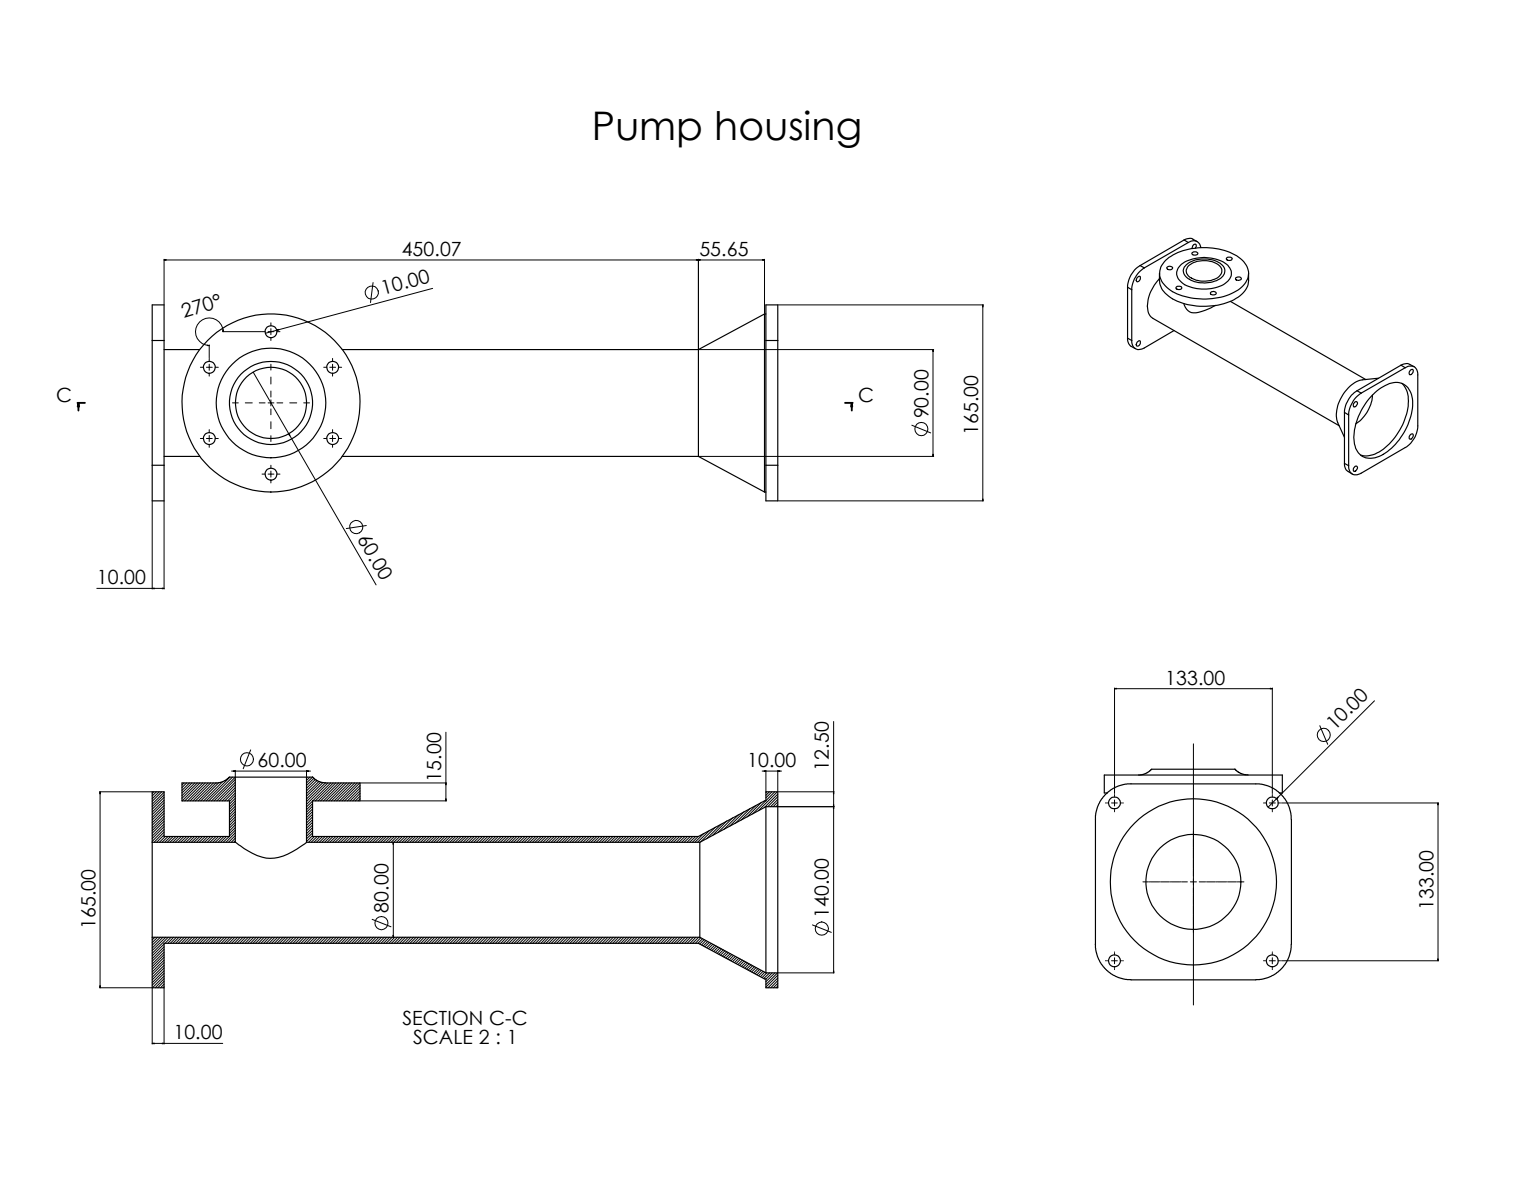
ISO-10303-21;
HEADER;
FILE_DESCRIPTION (('STEP AP214'),
    '1' );
FILE_NAME ('Pump housing.step',
    '2026-10-27T19:20:31',
    ( '' ),
    ( '' ),
    'SwSTEP 2.0',
    'SolidWorks 2025',
    '' );
FILE_SCHEMA (( 'AUTOMOTIVE_DESIGN' ));
ENDSEC;

DATA;
#8=( GEOMETRIC_REPRESENTATION_CONTEXT ( 3 ) GLOBAL_UNCERTAINTY_ASSIGNED_CONTEXT ( ( #20296 ) ) GLOBAL_UNIT_ASSIGNED_CONTEXT ( ( #22388, #16248, #14122 ) ) REPRESENTATION_CONTEXT ( 'NONE', 'WORKASPACE' ) );
#9=CARTESIAN_POINT ( 'NONE',  ( -200.0000000000000000, -52.49999999999992895, -52.49999999999999289 ) ) ;
#18=LINE ( 'NONE', #3258, #24208 ) ;
#20=CARTESIAN_POINT ( 'NONE',  ( -678.9461782662772293, 90.00000000000000000, 30.00000000000158096 ) ) ;
#22=DIRECTION ( 'NONE',  ( 0.000000000000000000, 0.000000000000000000, 1.000000000000000000 ) ) ;
#24=ORIENTED_EDGE ( 'NONE', *, *, #545, .T. ) ;
#40=DIRECTION ( 'NONE',  ( 0.000000000000000000, -0.000000000000000000, 1.000000000000000000 ) ) ;
#68=CARTESIAN_POINT ( 'NONE',  ( -210.0000000000000284, -52.49999999999991473, 82.49999999999998579 ) ) ;
#87=VERTEX_POINT ( 'NONE', #1727 ) ;
#102=DIRECTION ( 'NONE',  ( -1.000000000000000000, -1.836970198721030181E-16, 0.000000000000000000 ) ) ;
#143=DIRECTION ( 'NONE',  ( 0.000000000000000000, 1.000000000000000000, 0.000000000000000000 ) ) ;
#144=DIRECTION ( 'NONE',  ( 0.000000000000000000, 0.000000000000000000, 1.000000000000000000 ) ) ;
#153=DIRECTION ( 'NONE',  ( 1.000000000000000000, -0.000000000000000000, -0.000000000000000000 ) ) ;
#158=ORIENTED_EDGE ( 'NONE', *, *, #24110, .F. ) ;
#160=LINE ( 'NONE', #12392, #2622 ) ;
#170=CARTESIAN_POINT ( 'NONE',  ( -654.9559990268497813, 38.50095308322672594, 10.88967829900012418 ) ) ;
#178=CYLINDRICAL_SURFACE ( 'NONE', #9570, 69.99999999999998579 ) ;
#187=EDGE_LOOP ( 'NONE', ( #24603, #23674, #1863, #22741 ) ) ;
#188=ORIENTED_EDGE ( 'NONE', *, *, #14494, .T. ) ;
#231=AXIS2_PLACEMENT_3D ( 'NONE', #20688, #10567, #468 ) ;
#243=ORIENTED_EDGE ( 'NONE', *, *, #21209, .F. ) ;
#246=AXIS2_PLACEMENT_3D ( 'NONE', #22417, #6170, #12157 ) ;
#253=DIRECTION ( 'NONE',  ( 0.000000000000000000, 1.000000000000000000, 0.000000000000000000 ) ) ;
#254=DIRECTION ( 'NONE',  ( 0.000000000000000000, 0.000000000000000000, 1.000000000000000000 ) ) ;
#257=CIRCLE ( 'NONE', #21922, 30.00000000000000355 ) ;
#265=CIRCLE ( 'NONE', #15136, 44.99999999999997158 ) ;
#291=ADVANCED_FACE ( 'NONE', ( #12485 ), #392, .F. ) ;
#295=CIRCLE ( 'NONE', #24520, 34.99999999999999289 ) ;
#309=CARTESIAN_POINT ( 'NONE',  ( -655.7547062770219100, 39.08587256449166603, 8.516853268417087008 ) ) ;
#314=CIRCLE ( 'NONE', #24034, 5.000000000000011546 ) ;
#319=CARTESIAN_POINT ( 'NONE',  ( -661.6513161486427634, 44.74118846189777088, 4.856359999860261567 ) ) ;
#322=CIRCLE ( 'NONE', #24542, 5.000000000000004441 ) ;
#361=DIRECTION ( 'NONE',  ( 0.000000000000000000, 0.000000000000000000, 1.000000000000000000 ) ) ;
#383=ORIENTED_EDGE ( 'NONE', *, *, #7506, .F. ) ;
#392=CYLINDRICAL_SURFACE ( 'NONE', #8339, 5.000000000000007994 ) ;
#398=AXIS2_PLACEMENT_3D ( 'NONE', #8466, #22714, #5020 ) ;
#404=DIRECTION ( 'NONE',  ( 0.000000000000000000, 1.000000000000000000, 0.000000000000000000 ) ) ;
#408=LINE ( 'NONE', #4009, #2409 ) ;
#419=ORIENTED_EDGE ( 'NONE', *, *, #4206, .T. ) ;
#420=CARTESIAN_POINT ( 'NONE',  ( -726.9846540392142060, -66.50000000000001421, -66.50000000000005684 ) ) ;
#439=CIRCLE ( 'NONE', #14817, 44.99999999999997158 ) ;
#445=CARTESIAN_POINT ( 'NONE',  ( -650.6286843459992042, 35.47998694306583189, 18.48952057123083037 ) ) ;
#451=DIRECTION ( 'NONE',  ( 0.000000000000000000, 0.000000000000000000, -1.000000000000000000 ) ) ;
#455=CARTESIAN_POINT ( 'NONE',  ( -649.9764076924376468, 36.43131350046466821, 26.47907437413556053 ) ) ;
#462=DIRECTION ( 'NONE',  ( -1.000000000000000000, 0.000000000000000000, 0.000000000000000000 ) ) ;
#465=EDGE_CURVE ( 'NONE', #21399, #16736, #13986, .T. ) ;
#468=DIRECTION ( 'NONE',  ( 0.000000000000000000, 0.000000000000000000, 1.000000000000000000 ) ) ;
#472=DIRECTION ( 'NONE',  ( 0.000000000000000000, 0.000000000000000000, 1.000000000000000000 ) ) ;
#504=CARTESIAN_POINT ( 'NONE',  ( -726.9846540392142060, 52.49999999999986500, 82.49999999999998579 ) ) ;
#517=DIRECTION ( 'NONE',  ( 0.000000000000000000, 0.000000000000000000, 1.000000000000000000 ) ) ;
#526=DIRECTION ( 'NONE',  ( 0.000000000000000000, 0.000000000000000000, 1.000000000000000000 ) ) ;
#532=EDGE_CURVE ( 'NONE', #15801, #13855, #7476, .T. ) ;
#542=CARTESIAN_POINT ( 'NONE',  ( -597.4202930725263059, 39.67406997103029198, 5.193980993137010671 ) ) ;
#545=EDGE_CURVE ( 'NONE', #9566, #22711, #18550, .T. ) ;
#557=DIRECTION ( 'NONE',  ( 0.000000000000000000, 0.000000000000000000, 1.000000000000000000 ) ) ;
#567=VERTEX_POINT ( 'NONE', #26132 ) ;
#579=CARTESIAN_POINT ( 'NONE',  ( -656.5498746188114865, 39.67471111131991535, -5.189028119869940170 ) ) ;
#584=CARTESIAN_POINT ( 'NONE',  ( -265.6482238768269326, 0.000000000000000000, 0.000000000000000000 ) ) ;
#586=DIRECTION ( 'NONE',  ( 1.000000000000000000, 1.836970198721030427E-16, 0.000000000000000000 ) ) ;
#592=CARTESIAN_POINT ( 'NONE',  ( -611.2898122108906591, 32.33625437144371517, -31.30306668446011642 ) ) ;
#604=LINE ( 'NONE', #14430, #23210 ) ;
#609=DIRECTION ( 'NONE',  ( 0.000000000000000000, 0.000000000000000000, -1.000000000000000000 ) ) ;
#626=EDGE_CURVE ( 'NONE', #8935, #25083, #18123, .T. ) ;
#627=ORIENTED_EDGE ( 'NONE', *, *, #1350, .F. ) ;
#658=CARTESIAN_POINT ( 'NONE',  ( -678.9461782662772293, 75.00000000000000000, 35.00000000000159162 ) ) ;
#676=CARTESIAN_POINT ( 'NONE',  ( -716.9846540392142060, 66.50000000000009948, 61.50000000000005684 ) ) ;
#680=PLANE ( 'NONE',  #24960 ) ;
#685=FACE_OUTER_BOUND ( 'NONE', #11342, .T. ) ;
#687=EDGE_CURVE ( 'NONE', #14320, #23489, #997, .T. ) ;
#692=AXIS2_PLACEMENT_3D ( 'NONE', #22776, #2285, #14907 ) ;
#702=LINE ( 'NONE', #834, #8135 ) ;
#710=DIRECTION ( 'NONE',  ( 0.000000000000000000, 0.000000000000000000, -1.000000000000000000 ) ) ;
#713=DIRECTION ( 'NONE',  ( 0.000000000000000000, 0.000000000000000000, 1.000000000000000000 ) ) ;
#722=CARTESIAN_POINT ( 'NONE',  ( -661.7419054499291633, 44.81143869219462772, -4.158744080377950070 ) ) ;
#724=VECTOR ( 'NONE', #14723, 1000.000000000000000 ) ;
#728=CARTESIAN_POINT ( 'NONE',  ( -592.0657137250348114, 44.93697794005576185, -2.456499637838828853 ) ) ;
#740=CIRCLE ( 'NONE', #4985, 5.000000000000095035 ) ;
#749=DIRECTION ( 'NONE',  ( -1.000000000000000000, -1.836970198721030181E-16, 0.000000000000000000 ) ) ;
#758=ORIENTED_EDGE ( 'NONE', *, *, #3424, .F. ) ;
#770=DIRECTION ( 'NONE',  ( 0.000000000000000000, 1.000000000000000000, 0.000000000000000000 ) ) ;
#807=CARTESIAN_POINT ( 'NONE',  ( -617.0807177054949761, 28.23630110923742365, 28.33531756806318214 ) ) ;
#813=FACE_OUTER_BOUND ( 'NONE', #11620, .T. ) ;
#822=AXIS2_PLACEMENT_3D ( 'NONE', #9624, #3638, #5764 ) ;
#823=CARTESIAN_POINT ( 'NONE',  ( -678.9461782662789346, 90.00000000000000000, -24.99999999999826628 ) ) ;
#834=CARTESIAN_POINT ( 'NONE',  ( -678.9461782662772293, 75.00000000000000000, 25.00000000000157385 ) ) ;
#851=CARTESIAN_POINT ( 'NONE',  ( -642.7070543445415751, 32.34947999245193273, 31.28956669078001340 ) ) ;
#857=CARTESIAN_POINT ( 'NONE',  ( -592.4919920315402351, 44.60627086681392228, -6.055351194787411906 ) ) ;
#867=AXIS2_PLACEMENT_3D ( 'NONE', #5163, #9025, #21137 ) ;
#869=EDGE_CURVE ( 'NONE', #20514, #9693, #9078, .T. ) ;
#880=EDGE_CURVE ( 'NONE', #12353, #2322, #17250, .T. ) ;
#893=DIRECTION ( 'NONE',  ( -1.000000000000000000, -1.836970198721030181E-16, 0.000000000000000000 ) ) ;
#918=AXIS2_PLACEMENT_3D ( 'NONE', #25838, #19695, #3477 ) ;
#930=AXIS2_PLACEMENT_3D ( 'NONE', #26089, #1997, #5984 ) ;
#937=CARTESIAN_POINT ( 'NONE',  ( -605.2485198462496783, 34.24030537962636345, 20.68249523888561470 ) ) ;
#956=EDGE_LOOP ( 'NONE', ( #1715, #1989, #25855, #13026 ) ) ;
#958=CIRCLE ( 'NONE', #7716, 5.000000000000011546 ) ;
#978=LINE ( 'NONE', #16933, #23009 ) ;
#979=DIRECTION ( 'NONE',  ( 1.000000000000000000, -0.000000000000000000, -0.000000000000000000 ) ) ;
#987=CARTESIAN_POINT ( 'NONE',  ( -608.3670141342350917, 33.85940881687466231, 29.64264663930133992 ) ) ;
#997=B_SPLINE_CURVE_WITH_KNOTS ( 'NONE', 3,
 ( #7874, #1158, #13256, #1778, #9883, #26275, #12144, #15374, #24123, #5894, #14002, #10153, #20132, #21379, #25380, #22132, #21504, #3150, #7132, #15244, #23376, #12012, #5151, #11252, #19371, #3275, #9262, #17369, #25506, #7256, #23497, #579, #24530, #10410, #22405, #22927, #2713, #20665, #8149, #4438, #8686, #2301, #309, #6681, #170, #8411, #2177, #6159, #2573, #4708, #16264, #6418, #445, #4315, #24393, #16795, #12812, #18527, #12672, #18658, #4181, #16533, #18393, #8548, #14796, #10547, #6286, #12276, #20934, #24661, #14268, #18798, #14535, #22666 ),
 .UNSPECIFIED., .F., .F.,
 ( 4, 2, 2, 2, 2, 2, 2, 2, 2, 2, 2, 2, 2, 2, 2, 2, 2, 2, 2, 2, 2, 2, 2, 2, 2, 2, 2, 2, 2, 2, 2, 2, 2, 2, 2, 2, 4 ),
 ( 0.09798846907125773054, 0.09951654375267081354, 0.1010446184340838827, 0.1041007677969100348, 0.1071569171597361869, 0.1102130665225623529, 0.1132692158853885050, 0.1163253652482146572, 0.1224376639738672112, 0.1239657386552804053, 0.1254938133366935993, 0.1285499626995199873, 0.1346622614251727357, 0.1361903361065859297, 0.1377184107879991515, 0.1407745601508255950, 0.1438307095136520108, 0.1453587841950652049, 0.1468868588764783989, 0.1529991576021312305, 0.1545272322835444245, 0.1560553069649576186, 0.1591114563277840066, 0.1606395310091972561, 0.1621676056906105057, 0.1652237550534370325, 0.1682799044162635593, 0.1698079790976768089, 0.1713360537790900584, 0.1774483525047432786, 0.1805045018675699997, 0.1820325765489833603, 0.1835606512303967208, 0.1896729499560510512, 0.1927290993188783552, 0.1942571740002920211, 0.1957852486817056592 ),
 .UNSPECIFIED. ) ;
#1001=DIRECTION ( 'NONE',  ( -1.000000000000000000, 0.000000000000000000, 0.000000000000000000 ) ) ;
#1003=CARTESIAN_POINT ( 'NONE',  ( -626.9846540392142060, 90.00000000000000000, 0.000000000000000000 ) ) ;
#1004=LINE ( 'NONE', #19348, #9721 ) ;
#1045=ADVANCED_FACE ( 'NONE', ( #24084, #5858, #5998, #13964, #22099, #22760, #8115, #10649 ), #20625, .F. ) ;
#1079=ORIENTED_EDGE ( 'NONE', *, *, #14192, .F. ) ;
#1081=DIRECTION ( 'NONE',  ( -1.836970198721030427E-16, 1.000000000000000000, -1.321694076934715579E-16 ) ) ;
#1087=CARTESIAN_POINT ( 'NONE',  ( -716.9846540392142060, 66.50000000000009948, -61.50000000000004974 ) ) ;
#1089=CARTESIAN_POINT ( 'NONE',  ( -626.9846540392142060, 75.00000000000000000, -54.99999999999995026 ) ) ;
#1094=DIRECTION ( 'NONE',  ( 0.000000000000000000, 0.000000000000000000, 1.000000000000000000 ) ) ;
#1100=CARTESIAN_POINT ( 'NONE',  ( 0.000000000000000000, 0.000000000000000000, 0.000000000000000000 ) ) ;
#1103=AXIS2_PLACEMENT_3D ( 'NONE', #2737, #10842, #13228 ) ;
#1107=CARTESIAN_POINT ( 'NONE',  ( -626.9846540392142060, 75.00000000000000000, -65.00000000000004263 ) ) ;
#1116=CYLINDRICAL_SURFACE ( 'NONE', #8150, 44.99999999999997158 ) ;
#1118=EDGE_LOOP ( 'NONE', ( #10707, #11181, #17708, #25036 ) ) ;
#1123=CIRCLE ( 'NONE', #20660, 39.99999999999997158 ) ;
#1126=EDGE_CURVE ( 'NONE', #8002, #9153, #408, .T. ) ;
#1139=LINE ( 'NONE', #17860, #8300 ) ;
#1145=AXIS2_PLACEMENT_3D ( 'NONE', #16360, #16231, #22372 ) ;
#1152=CIRCLE ( 'NONE', #8804, 29.99999999999999289 ) ;
#1158=CARTESIAN_POINT ( 'NONE',  ( -627.5027443299393326, 26.45751311064577038, -30.00000000000005329 ) ) ;
#1177=LINE ( 'NONE', #21004, #23952 ) ;
#1180=VERTEX_POINT ( 'NONE', #10214 ) ;
#1184=CARTESIAN_POINT ( 'NONE',  ( 0.000000000000000000, 0.000000000000000000, 0.000000000000000000 ) ) ;
#1188=DIRECTION ( 'NONE',  ( 1.000000000000000000, -0.000000000000000000, -0.000000000000000000 ) ) ;
#1193=CARTESIAN_POINT ( 'NONE',  ( -598.6670741908344553, 38.75362502970266121, -9.956152867874221712 ) ) ;
#1200=EDGE_CURVE ( 'NONE', #17385, #7220, #19400, .T. ) ;
#1202=ORIENTED_EDGE ( 'NONE', *, *, #1431, .T. ) ;
#1213=ORIENTED_EDGE ( 'NONE', *, *, #19964, .F. ) ;
#1239=FACE_OUTER_BOUND ( 'NONE', #12293, .T. ) ;
#1240=CARTESIAN_POINT ( 'NONE',  ( -614.3062485512364219, 30.98201105461428995, 32.64211941558109942 ) ) ;
#1266=DIRECTION ( 'NONE',  ( -1.000000000000000000, 0.000000000000000000, 0.000000000000000000 ) ) ;
#1274=FACE_OUTER_BOUND ( 'NONE', #4173, .T. ) ;
#1282=AXIS2_PLACEMENT_3D ( 'NONE', #20, #15834, #6140 ) ;
#1310=CARTESIAN_POINT ( 'NONE',  ( -626.9846540392142060, 75.00000000000000000, 0.000000000000000000 ) ) ;
#1315=CARTESIAN_POINT ( 'NONE',  ( -611.8146452038604366, 30.48906968622233649, -25.89952525135564798 ) ) ;
#1336=VERTEX_POINT ( 'NONE', #11014 ) ;
#1337=EDGE_CURVE ( 'NONE', #2862, #11180, #19124, .T. ) ;
#1338=VERTEX_POINT ( 'NONE', #8746 ) ;
#1343=AXIS2_PLACEMENT_3D ( 'NONE', #16929, #25063, #6815 ) ;
#1350=EDGE_CURVE ( 'NONE', #16014, #12649, #10884, .T. ) ;
#1366=CARTESIAN_POINT ( 'NONE',  ( -639.6467708969067871, 30.97534985185962242, -32.64842303514383559 ) ) ;
#1375=FACE_OUTER_BOUND ( 'NONE', #4952, .T. ) ;
#1386=DIRECTION ( 'NONE',  ( 1.000000000000000000, -0.000000000000000000, -0.000000000000000000 ) ) ;
#1398=DIRECTION ( 'NONE',  ( 0.000000000000000000, -1.000000000000000000, 0.000000000000000000 ) ) ;
#1401=ORIENTED_EDGE ( 'NONE', *, *, #19720, .F. ) ;
#1431=EDGE_CURVE ( 'NONE', #11418, #14640, #18510, .T. ) ;
#1432=ORIENTED_EDGE ( 'NONE', *, *, #16631, .F. ) ;
#1461=ORIENTED_EDGE ( 'NONE', *, *, #4114, .T. ) ;
#1463=DIRECTION ( 'NONE',  ( 1.000000000000000000, 1.836970198721030427E-16, -0.000000000000000000 ) ) ;
#1470=LINE ( 'NONE', #1089, #20851 ) ;
#1473=DIRECTION ( 'NONE',  ( 1.000000000000000000, -0.000000000000000000, -0.000000000000000000 ) ) ;
#1490=ORIENTED_EDGE ( 'NONE', *, *, #16234, .F. ) ;
#1492=EDGE_CURVE ( 'NONE', #12353, #7498, #10988, .T. ) ;
#1493=DIRECTION ( 'NONE',  ( -1.000000000000000000, -1.836970198721030181E-16, 0.000000000000000000 ) ) ;
#1494=CARTESIAN_POINT ( 'NONE',  ( -615.3642883616319068, 30.56114224079260211, 33.03453977807346575 ) ) ;
#1496=CARTESIAN_POINT ( 'NONE',  ( -265.6482238768269326, 4.898587196589409870E-15, 39.99999999999997158 ) ) ;
#1503=ORIENTED_EDGE ( 'NONE', *, *, #5754, .F. ) ;
#1515=DIRECTION ( 'NONE',  ( 0.000000000000000000, 0.000000000000000000, -1.000000000000000000 ) ) ;
#1529=ADVANCED_FACE ( 'NONE', ( #17473 ), #21477, .F. ) ;
#1531=EDGE_LOOP ( 'NONE', ( #6366, #4909, #3109, #25138 ) ) ;
#1533=VECTOR ( 'NONE', #12308, 1000.000000000000000 ) ;
#1548=AXIS2_PLACEMENT_3D ( 'NONE', #18108, #1759, #22118 ) ;
#1559=ORIENTED_EDGE ( 'NONE', *, *, #25834, .T. ) ;
#1564=VERTEX_POINT ( 'NONE', #25870 ) ;
#1586=CARTESIAN_POINT ( 'NONE',  ( -210.0000000000000284, 66.50000000000009948, 66.50000000000005684 ) ) ;
#1593=VERTEX_POINT ( 'NONE', #3641 ) ;
#1596=VERTEX_POINT ( 'NONE', #23600 ) ;
#1599=ORIENTED_EDGE ( 'NONE', *, *, #18731, .T. ) ;
#1601=DIRECTION ( 'NONE',  ( -1.000000000000000000, 0.000000000000000000, 0.000000000000000000 ) ) ;
#1630=ORIENTED_EDGE ( 'NONE', *, *, #20692, .F. ) ;
#1639=CARTESIAN_POINT ( 'NONE',  ( -210.0000000000000284, -61.50000000000002132, -66.50000000000005684 ) ) ;
#1651=CARTESIAN_POINT ( 'NONE',  ( -626.9846540392142060, 95.00000000000000000, 30.00000000000005329 ) ) ;
#1652=DIRECTION ( 'NONE',  ( -1.000000000000000000, -1.836970198721030181E-16, 0.000000000000000000 ) ) ;
#1668=EDGE_CURVE ( 'NONE', #12661, #21773, #1139, .T. ) ;
#1678=DIRECTION ( 'NONE',  ( 1.000000000000000000, -0.000000000000000000, -0.000000000000000000 ) ) ;
#1684=CARTESIAN_POINT ( 'NONE',  ( -210.0000000000000284, 66.50000000000009948, 66.50000000000005684 ) ) ;
#1692=ORIENTED_EDGE ( 'NONE', *, *, #20350, .T. ) ;
#1708=CARTESIAN_POINT ( 'NONE',  ( -604.5625608938773894, 34.67764305556000437, -19.95380784793596973 ) ) ;
#1715=ORIENTED_EDGE ( 'NONE', *, *, #626, .F. ) ;
#1721=VERTEX_POINT ( 'NONE', #26011 ) ;
#1727=CARTESIAN_POINT ( 'NONE',  ( -265.6482238768269326, 0.000000000000000000, -39.99999999999997158 ) ) ;
#1746=CARTESIAN_POINT ( 'NONE',  ( -716.9846540392142060, 52.49999999999991473, -82.49999999999998579 ) ) ;
#1753=EDGE_LOOP ( 'NONE', ( #10197, #3904, #12389, #11955 ) ) ;
#1757=CARTESIAN_POINT ( 'NONE',  ( -716.9846540392142060, 52.50000000000007816, -52.49999999999999289 ) ) ;
#1759=DIRECTION ( 'NONE',  ( 0.000000000000000000, 1.000000000000000000, 0.000000000000000000 ) ) ;
#1760=VERTEX_POINT ( 'NONE', #1651 ) ;
#1761=CIRCLE ( 'NONE', #7270, 30.00000000000000355 ) ;
#1767=ORIENTED_EDGE ( 'NONE', *, *, #12722, .F. ) ;
#1777=CYLINDRICAL_SURFACE ( 'NONE', #3646, 5.000000000000011546 ) ;
#1778=CARTESIAN_POINT ( 'NONE',  ( -629.0557304578984485, 26.53345902544097967, -29.93287798360601570 ) ) ;
#1797=ORIENTED_EDGE ( 'NONE', *, *, #5393, .F. ) ;
#1825=EDGE_LOOP ( 'NONE', ( #17662, #23179 ) ) ;
#1850=DIRECTION ( 'NONE',  ( 0.000000000000000000, -1.000000000000000000, 0.000000000000000000 ) ) ;
#1852=ORIENTED_EDGE ( 'NONE', *, *, #12545, .T. ) ;
#1863=ORIENTED_EDGE ( 'NONE', *, *, #1350, .T. ) ;
#1868=CARTESIAN_POINT ( 'NONE',  ( -726.9846540392142060, 66.50000000000009948, 61.50000000000005684 ) ) ;
#1880=DIRECTION ( 'NONE',  ( 0.000000000000000000, 1.000000000000000000, 0.000000000000000000 ) ) ;
#1890=DIRECTION ( 'NONE',  ( 0.000000000000000000, 0.000000000000000000, -1.000000000000000000 ) ) ;
#1895=( NAMED_UNIT ( * ) SI_UNIT ( $, .STERADIAN. ) SOLID_ANGLE_UNIT ( ) );
#1897=ORIENTED_EDGE ( 'NONE', *, *, #626, .T. ) ;
#1910=CARTESIAN_POINT ( 'NONE',  ( -626.9846540392142060, 75.00000000000000000, -74.99999999999991473 ) ) ;
#1916=DIRECTION ( 'NONE',  ( 0.000000000000000000, 0.000000000000000000, 1.000000000000000000 ) ) ;
#1921=CARTESIAN_POINT ( 'NONE',  ( -678.9461782662789346, 75.00000000000000000, -24.99999999999826628 ) ) ;
#1928=ORIENTED_EDGE ( 'NONE', *, *, #25834, .F. ) ;
#1955=AXIS2_PLACEMENT_3D ( 'NONE', #23408, #21788, #23653 ) ;
#1962=VECTOR ( 'NONE', #14925, 1000.000000000000000 ) ;
#1988=EDGE_LOOP ( 'NONE', ( #758, #21990, #4423, #14129 ) ) ;
#1989=ORIENTED_EDGE ( 'NONE', *, *, #16482, .T. ) ;
#1997=DIRECTION ( 'NONE',  ( -1.000000000000000000, 0.000000000000000000, 0.000000000000000000 ) ) ;
#2000=AXIS2_PLACEMENT_3D ( 'NONE', #23417, #23537, #25292 ) ;
#2019=LINE ( 'NONE', #4153, #21289 ) ;
#2030=DIRECTION ( 'NONE',  ( -1.000000000000000000, 0.000000000000000000, 0.000000000000000000 ) ) ;
#2041=CARTESIAN_POINT ( 'NONE',  ( -199.9999999999999716, -82.49999999999991473, -52.49999999999977973 ) ) ;
#2049=CARTESIAN_POINT ( 'NONE',  ( -716.9846540392142060, 82.50000000000008527, 52.49999999999980105 ) ) ;
#2054=LINE ( 'NONE', #16410, #18940 ) ;
#2064=ORIENTED_EDGE ( 'NONE', *, *, #22985, .T. ) ;
#2065=ORIENTED_EDGE ( 'NONE', *, *, #22233, .F. ) ;
#2077=LINE ( 'NONE', #4214, #17372 ) ;
#2081=LINE ( 'NONE', #16303, #1533 ) ;
#2094=ORIENTED_EDGE ( 'NONE', *, *, #16482, .F. ) ;
#2102=CARTESIAN_POINT ( 'NONE',  ( -575.0231298121445889, 75.00000000000000000, 29.99999999999825206 ) ) ;
#2118=PRODUCT_CONTEXT ( 'NONE', #10201, 'mechanical' ) ;
#2123=ORIENTED_EDGE ( 'NONE', *, *, #23092, .F. ) ;
#2139=DIRECTION ( 'NONE',  ( 1.000000000000000000, 1.836970198721030427E-16, -0.000000000000000000 ) ) ;
#2143=FACE_BOUND ( 'NONE', #4565, .T. ) ;
#2144=AXIS2_PLACEMENT_3D ( 'NONE', #13336, #11585, #19580 ) ;
#2152=VERTEX_POINT ( 'NONE', #16029 ) ;
#2154=FACE_OUTER_BOUND ( 'NONE', #25295, .T. ) ;
#2163=DIRECTION ( 'NONE',  ( 0.8802361161597900274, 0.000000000000000000, -0.4745359626076074422 ) ) ;
#2165=ADVANCED_FACE ( 'NONE', ( #7613 ), #14146, .F. ) ;
#2171=EDGE_CURVE ( 'NONE', #24112, #7498, #20193, .T. ) ;
#2172=ADVANCED_FACE ( 'NONE', ( #22935 ), #6425, .F. ) ;
#2177=CARTESIAN_POINT ( 'NONE',  ( -654.1659037529333318, 37.93148257888354635, 12.70525021040782754 ) ) ;
#2180=DIRECTION ( 'NONE',  ( -1.000000000000000000, 0.000000000000000000, 0.000000000000000000 ) ) ;
#2187=FACE_BOUND ( 'NONE', #25625, .T. ) ;
#2198=ORIENTED_EDGE ( 'NONE', *, *, #19384, .F. ) ;
#2204=FACE_OUTER_BOUND ( 'NONE', #13398, .T. ) ;
#2205=CARTESIAN_POINT ( 'NONE',  ( -726.9846540392142060, -52.49999999999991473, 82.49999999999998579 ) ) ;
#2227=DIRECTION ( 'NONE',  ( -1.000000000000000000, -1.836970198721030181E-16, 0.000000000000000000 ) ) ;
#2247=ORIENTED_EDGE ( 'NONE', *, *, #16442, .F. ) ;
#2252=EDGE_CURVE ( 'NONE', #6112, #5576, #6594, .T. ) ;
#2257=EDGE_LOOP ( 'NONE', ( #16312, #18069, #19048, #6656 ) ) ;
#2285=DIRECTION ( 'NONE',  ( -1.000000000000000000, 0.000000000000000000, 0.000000000000000000 ) ) ;
#2301=CARTESIAN_POINT ( 'NONE',  ( -655.8941833601360258, 39.18869065112085082, 8.031053782042897993 ) ) ;
#2311=CARTESIAN_POINT ( 'NONE',  ( -660.6855337863669320, 43.99654503343406020, 9.519970529664389502 ) ) ;
#2322=VERTEX_POINT ( 'NONE', #4715 ) ;
#2340=ADVANCED_FACE ( 'NONE', ( #12819 ), #178, .F. ) ;
#2387=VERTEX_POINT ( 'NONE', #24941 ) ;
#2404=EDGE_CURVE ( 'NONE', #1338, #2553, #2054, .T. ) ;
#2405=CARTESIAN_POINT ( 'NONE',  ( -716.9846540392142060, -52.49999999999992895, -52.49999999999999289 ) ) ;
#2409=VECTOR ( 'NONE', #2139, 1000.000000000000000 ) ;
#2410=FACE_OUTER_BOUND ( 'NONE', #20252, .T. ) ;
#2432=DIRECTION ( 'NONE',  ( 0.000000000000000000, 1.000000000000000000, 0.000000000000000000 ) ) ;
#2449=CARTESIAN_POINT ( 'NONE',  ( -592.4863246237233625, 44.61088836317698281, 5.935200987246425974 ) ) ;
#2453=DIRECTION ( 'NONE',  ( 0.000000000000000000, -1.000000000000000000, 0.000000000000000000 ) ) ;
#2482=ADVANCED_FACE ( 'NONE', ( #24803 ), #2580, .F. ) ;
#2499=DIRECTION ( 'NONE',  ( 0.000000000000000000, 1.000000000000000000, 0.000000000000000000 ) ) ;
#2518=ORIENTED_EDGE ( 'NONE', *, *, #3123, .F. ) ;
#2520=DIRECTION ( 'NONE',  ( 0.000000000000000000, 1.000000000000000000, 0.000000000000000000 ) ) ;
#2533=CARTESIAN_POINT ( 'NONE',  ( -598.0968614159205572, 39.17219949141968272, 8.155532079469960394 ) ) ;
#2546=DIRECTION ( 'NONE',  ( 0.000000000000000000, 0.000000000000000000, 1.000000000000000000 ) ) ;
#2548=AXIS2_PLACEMENT_3D ( 'NONE', #23606, #16375, #12123 ) ;
#2553=VERTEX_POINT ( 'NONE', #8910 ) ;
#2558=ORIENTED_EDGE ( 'NONE', *, *, #9614, .T. ) ;
#2568=DIRECTION ( 'NONE',  ( 0.000000000000000000, 1.000000000000000000, 0.000000000000000000 ) ) ;
#2573=CARTESIAN_POINT ( 'NONE',  ( -653.5054087259286462, 37.46094337825315534, 14.03175942970671386 ) ) ;
#2580=CYLINDRICAL_SURFACE ( 'NONE', #25729, 4.999999999999962697 ) ;
#2582=CARTESIAN_POINT ( 'NONE',  ( -653.4170159849278434, 38.71178713871361765, 22.94860588273028768 ) ) ;
#2587=CARTESIAN_POINT ( 'NONE',  ( -595.8093182457012063, 42.09229316366772622, 15.94989993472014511 ) ) ;
#2588=ORIENTED_EDGE ( 'NONE', *, *, #25417, .F. ) ;
#2592=DIRECTION ( 'NONE',  ( 1.000000000000000000, 1.836970198721030427E-16, -0.000000000000000000 ) ) ;
#2594=AXIS2_PLACEMENT_3D ( 'NONE', #23312, #23060, #22792 ) ;
#2597=DIRECTION ( 'NONE',  ( 0.000000000000000000, 0.000000000000000000, 1.000000000000000000 ) ) ;
#2609=CARTESIAN_POINT ( 'NONE',  ( -575.0231298121445889, 75.00000000000000000, 24.99999999999828759 ) ) ;
#2622=VECTOR ( 'NONE', #11998, 1000.000000000000000 ) ;
#2625=ORIENTED_EDGE ( 'NONE', *, *, #7357, .F. ) ;
#2664=AXIS2_PLACEMENT_3D ( 'NONE', #2981, #19204, #3354 ) ;
#2676=CARTESIAN_POINT ( 'NONE',  ( -619.9449226945228020, 27.37410191665372494, 29.16662018060867112 ) ) ;
#2694=FACE_BOUND ( 'NONE', #25987, .T. ) ;
#2696=ORIENTED_EDGE ( 'NONE', *, *, #3076, .F. ) ;
#2699=DIRECTION ( 'NONE',  ( 0.000000000000000000, 1.000000000000000000, 0.000000000000000000 ) ) ;
#2702=ORIENTED_EDGE ( 'NONE', *, *, #4106, .F. ) ;
#2713=CARTESIAN_POINT ( 'NONE',  ( -656.9835591184084933, 39.99917881009967147, -0.5754573772625048989 ) ) ;
#2722=CARTESIAN_POINT ( 'NONE',  ( -661.9203515605751136, 44.94993422606702893, 2.443437321343243429 ) ) ;
#2726=CARTESIAN_POINT ( 'NONE',  ( -595.8013259146971450, 42.09546181640034490, -16.06146874878389141 ) ) ;
#2733=ORIENTED_EDGE ( 'NONE', *, *, #6809, .T. ) ;
#2737=CARTESIAN_POINT ( 'NONE',  ( -210.0000000000000284, -52.49999999999991473, 52.49999999999999289 ) ) ;
#2751=ADVANCED_FACE ( 'NONE', ( #22759 ), #8510, .F. ) ;
#2754=DIRECTION ( 'NONE',  ( 0.000000000000000000, 0.000000000000000000, 1.000000000000000000 ) ) ;
#2765=CARTESIAN_POINT ( 'NONE',  ( 0.000000000000000000, 0.000000000000000000, -75.00000000000000000 ) ) ;
#2781=CYLINDRICAL_SURFACE ( 'NONE', #11057, 4.999999999999997335 ) ;
#2806=CARTESIAN_POINT ( 'NONE',  ( -622.8837209345899737, 26.70509413432482049, 29.78579685810782252 ) ) ;
#2809=AXIS2_PLACEMENT_3D ( 'NONE', #1003, #18966, #22694 ) ;
#2825=ORIENTED_EDGE ( 'NONE', *, *, #22824, .F. ) ;
#2842=EDGE_CURVE ( 'NONE', #5576, #15935, #17400, .T. ) ;
#2857=CIRCLE ( 'NONE', #22396, 15.00000000000000000 ) ;
#2858=ORIENTED_EDGE ( 'NONE', *, *, #9722, .F. ) ;
#2861=CARTESIAN_POINT ( 'NONE',  ( -603.9616649909638681, 36.45097493161564728, 26.45255915120217693 ) ) ;
#2862=VERTEX_POINT ( 'NONE', #15654 ) ;
#2864=DIRECTION ( 'NONE',  ( 0.000000000000000000, 1.000000000000000000, 0.000000000000000000 ) ) ;
#2867=ORIENTED_EDGE ( 'NONE', *, *, #19308, .F. ) ;
#2873=DIRECTION ( 'NONE',  ( -0.000000000000000000, 1.000000000000000000, -0.000000000000000000 ) ) ;
#2880=CARTESIAN_POINT ( 'NONE',  ( -200.0000000000000000, -66.50000000000001421, -66.50000000000005684 ) ) ;
#2899=EDGE_CURVE ( 'NONE', #2983, #16736, #10016, .T. ) ;
#2912=FACE_OUTER_BOUND ( 'NONE', #21555, .T. ) ;
#2915=VERTEX_POINT ( 'NONE', #23778 ) ;
#2942=ORIENTED_EDGE ( 'NONE', *, *, #9722, .T. ) ;
#2947=AXIS2_PLACEMENT_3D ( 'NONE', #6165, #26280, #1916 ) ;
#2950=EDGE_LOOP ( 'NONE', ( #17042, #10599, #1432, #9437 ) ) ;
#2951=EDGE_LOOP ( 'NONE', ( #2702, #19675, #20637, #14350 ) ) ;
#2962=LINE ( 'NONE', #21056, #3828 ) ;
#2970=ADVANCED_FACE ( 'NONE', ( #25664 ), #17526, .T. ) ;
#2971=VECTOR ( 'NONE', #12257, 1000.000000000000000 ) ;
#2976=CARTESIAN_POINT ( 'NONE',  ( -645.5897708877611194, 33.84656210914351959, -29.66564330929828230 ) ) ;
#2981=CARTESIAN_POINT ( 'NONE',  ( -716.9846540392142060, -66.50000000000001421, 66.50000000000005684 ) ) ;
#2982=CARTESIAN_POINT ( 'NONE',  ( -596.9048215538962268, 41.27960141593418797, -18.03334258849684701 ) ) ;
#2983=VERTEX_POINT ( 'NONE', #7410 ) ;
#2987=ADVANCED_FACE ( 'NONE', ( #7162 ), #15524, .T. ) ;
#2988=CARTESIAN_POINT ( 'NONE',  ( 0.000000000000000000, 0.000000000000000000, 0.000000000000000000 ) ) ;
#2996=LINE ( 'NONE', #20826, #10015 ) ;
#3008=AXIS2_PLACEMENT_3D ( 'NONE', #5611, #15208, #23458 ) ;
#3020=DIRECTION ( 'NONE',  ( 0.000000000000000000, 0.000000000000000000, 1.000000000000000000 ) ) ;
#3030=CARTESIAN_POINT ( 'NONE',  ( 0.000000000000000000, 9.184850993605148733E-15, 75.00000000000000000 ) ) ;
#3038=VECTOR ( 'NONE', #12658, 1000.000000000000000 ) ;
#3045=EDGE_LOOP ( 'NONE', ( #5456, #12790, #12055, #22189 ) ) ;
#3057=CARTESIAN_POINT ( 'NONE',  ( -210.0000000000000284, 0.000000000000000000, 0.000000000000000000 ) ) ;
#3060=CARTESIAN_POINT ( 'NONE',  ( -599.0758207628625769, 38.45631679711321738, 11.01587919049791076 ) ) ;
#3068=CARTESIAN_POINT ( 'NONE',  ( -716.9846540392142060, 66.50000000000009948, -66.50000000000005684 ) ) ;
#3073=CYLINDRICAL_SURFACE ( 'NONE', #6053, 5.000000000000004441 ) ;
#3076=EDGE_CURVE ( 'NONE', #23087, #10307, #2081, .T. ) ;
#3080=EDGE_LOOP ( 'NONE', ( #9441, #19397, #23709, #22220 ) ) ;
#3092=CARTESIAN_POINT ( 'NONE',  ( -716.9846540392142060, -82.49999999999991473, -52.49999999999977973 ) ) ;
#3103=CARTESIAN_POINT ( 'NONE',  ( -638.5875168204022430, 30.55437902294503161, -33.04080401100450359 ) ) ;
#3108=CARTESIAN_POINT ( 'NONE',  ( -617.0039382655427289, 29.98920333220143419, 33.55165781079447385 ) ) ;
#3109=ORIENTED_EDGE ( 'NONE', *, *, #9480, .F. ) ;
#3113=VERTEX_POINT ( 'NONE', #16438 ) ;
#3117=CARTESIAN_POINT ( 'NONE',  ( 0.000000000000000000, 0.000000000000000000, -44.99999999999997158 ) ) ;
#3120=DIRECTION ( 'NONE',  ( 0.000000000000000000, 0.000000000000000000, 1.000000000000000000 ) ) ;
#3123=EDGE_CURVE ( 'NONE', #21007, #20921, #20037, .T. ) ;
#3150=CARTESIAN_POINT ( 'NONE',  ( -648.4009115869816924, 34.03803227582063329, -21.01344779086421255 ) ) ;
#3151=EDGE_CURVE ( 'NONE', #1593, #6964, #20646, .T. ) ;
#3157=DIRECTION ( 'NONE',  ( 1.000000000000000000, -0.000000000000000000, -0.000000000000000000 ) ) ;
#3167=VERTEX_POINT ( 'NONE', #14039 ) ;
#3172=EDGE_LOOP ( 'NONE', ( #6273, #9609 ) ) ;
#3184=CARTESIAN_POINT ( 'NONE',  ( -598.2148974052754511, 39.08565501426862454, -8.517844816818030296 ) ) ;
#3203=CIRCLE ( 'NONE', #231, 5.000000000000039080 ) ;
#3224=AXIS2_PLACEMENT_3D ( 'NONE', #4997, #18960, #3120 ) ;
#3228=DIRECTION ( 'NONE',  ( -1.000000000000000000, 0.000000000000000000, 0.000000000000000000 ) ) ;
#3233=EDGE_LOOP ( 'NONE', ( #18372, #13913, #1559, #22423 ) ) ;
#3236=DIRECTION ( 'NONE',  ( -1.000000000000000000, -1.836970198721030181E-16, 0.000000000000000000 ) ) ;
#3238=ORIENTED_EDGE ( 'NONE', *, *, #25270, .F. ) ;
#3242=DIRECTION ( 'NONE',  ( 1.000000000000000000, 1.836970198721030427E-16, -0.000000000000000000 ) ) ;
#3243=CLOSED_SHELL ( 'NONE', ( #11757, #22727, #20867, #12476, #10434, #24263, #18492, #1529, #17565, #25370, #17208, #15951, #19396, #10881, #11280, #23525, #18081, #23913, #20057, #3963, #2165, #20870, #12486, #18771, #24445, #5556, #12232, #14264, #14679, #12482, #25042, #20355, #2970, #9287, #20548, #2172, #2987, #2751, #2340, #16882, #17246, #24951, #21636, #15474, #13245, #14824, #11974, #22263, #19247, #1045, #5863, #291, #2482, #7282, #5025, #6375, #9946, #4875, #5328, #14432, #8067, #4219, #9376, #10598, #17893, #12575, #9237, #14345, #24209, #24635, #22975 ) ) ;
#3244=DIRECTION ( 'NONE',  ( 0.000000000000000000, 0.000000000000000000, -1.000000000000000000 ) ) ;
#3258=CARTESIAN_POINT ( 'NONE',  ( -716.9846540392142060, -82.49999999999991473, 52.49999999999977263 ) ) ;
#3275=CARTESIAN_POINT ( 'NONE',  ( -654.7090520960496178, 38.32262798275520055, -11.47173633207906107 ) ) ;
#3312=CARTESIAN_POINT ( 'NONE',  ( -614.8060072283433328, 29.12309729869464192, -27.42103544326355546 ) ) ;
#3328=CARTESIAN_POINT ( 'NONE',  ( -678.9461782662772293, 75.00000000000000000, 30.00000000000158096 ) ) ;
#3330=ORIENTED_EDGE ( 'NONE', *, *, #18880, .T. ) ;
#3337=CARTESIAN_POINT ( 'NONE',  ( -210.0000000000000284, 0.000000000000000000, -75.00000000000000000 ) ) ;
#3345=AXIS2_PLACEMENT_3D ( 'NONE', #7445, #17435, #11438 ) ;
#3354=DIRECTION ( 'NONE',  ( 0.000000000000000000, 0.000000000000000000, 1.000000000000000000 ) ) ;
#3356=EDGE_LOOP ( 'NONE', ( #20075, #16422, #24649, #24167 ) ) ;
#3363=EDGE_CURVE ( 'NONE', #5576, #6112, #18528, .T. ) ;
#3378=DIRECTION ( 'NONE',  ( -1.000000000000000000, 0.000000000000000000, 0.000000000000000000 ) ) ;
#3390=AXIS2_PLACEMENT_3D ( 'NONE', #10930, #24638, #6792 ) ;
#3398=CYLINDRICAL_SURFACE ( 'NONE', #20716, 74.99999999999991473 ) ;
#3410=FACE_OUTER_BOUND ( 'NONE', #2257, .T. ) ;
#3415=ORIENTED_EDGE ( 'NONE', *, *, #11169, .T. ) ;
#3424=EDGE_CURVE ( 'NONE', #13855, #17045, #25460, .T. ) ;
#3425=CARTESIAN_POINT ( 'NONE',  ( -626.9846540392142060, 75.00000000000000000, 34.99999999999999289 ) ) ;
#3427=EDGE_CURVE ( 'NONE', #24064, #13093, #257, .T. ) ;
#3428=FACE_OUTER_BOUND ( 'NONE', #4333, .T. ) ;
#3434=CYLINDRICAL_SURFACE ( 'NONE', #13021, 29.99999999999999645 ) ;
#3435=CARTESIAN_POINT ( 'NONE',  ( -622.8776819133570370, 26.70401283558588901, -29.78701626806179092 ) ) ;
#3439=AXIS2_PLACEMENT_3D ( 'NONE', #18849, #2227, #25239 ) ;
#3442=AXIS2_PLACEMENT_3D ( 'NONE', #9692, #3450, #25808 ) ;
#3444=AXIS2_PLACEMENT_3D ( 'NONE', #3731, #1473, #7571 ) ;
#3450=DIRECTION ( 'NONE',  ( -1.000000000000000000, -1.836970198721030181E-16, 0.000000000000000000 ) ) ;
#3455=DIRECTION ( 'NONE',  ( 1.000000000000000000, 1.836970198721030427E-16, -0.000000000000000000 ) ) ;
#3463=CARTESIAN_POINT ( 'NONE',  ( -210.0000000000000284, 82.50000000000008527, -52.49999999999978684 ) ) ;
#3477=DIRECTION ( 'NONE',  ( 0.000000000000000000, 0.000000000000000000, -1.000000000000000000 ) ) ;
#3500=AXIS2_PLACEMENT_3D ( 'NONE', #9344, #7214, #17198 ) ;
#3520=ORIENTED_EDGE ( 'NONE', *, *, #10207, .F. ) ;
#3527=CARTESIAN_POINT ( 'NONE',  ( -716.9846540392142060, 52.49999999999986500, 82.49999999999998579 ) ) ;
#3557=CARTESIAN_POINT ( 'NONE',  ( -626.9846540392142060, 75.00000000000000000, -60.00000000000000000 ) ) ;
#3571=VERTEX_POINT ( 'NONE', #11332 ) ;
#3578=VERTEX_POINT ( 'NONE', #23331 ) ;
#3579=FACE_OUTER_BOUND ( 'NONE', #18647, .T. ) ;
#3581=ORIENTED_EDGE ( 'NONE', *, *, #17434, .T. ) ;
#3626=EDGE_CURVE ( 'NONE', #17304, #7651, #19784, .T. ) ;
#3635=DIRECTION ( 'NONE',  ( 0.000000000000000000, 0.000000000000000000, 1.000000000000000000 ) ) ;
#3638=DIRECTION ( 'NONE',  ( -1.000000000000000000, -1.836970198721030181E-16, 0.000000000000000000 ) ) ;
#3641=CARTESIAN_POINT ( 'NONE',  ( -716.9846540392142060, -66.50000000000001421, -71.50000000000005684 ) ) ;
#3646=AXIS2_PLACEMENT_3D ( 'NONE', #3911, #15850, #6030 ) ;
#3653=CARTESIAN_POINT ( 'NONE',  ( -626.9846540392097722, 75.00000000000000000, 59.99999999999999289 ) ) ;
#3673=DIRECTION ( 'NONE',  ( 0.000000000000000000, -1.000000000000000000, 0.000000000000000000 ) ) ;
#3694=DIRECTION ( 'NONE',  ( 1.000000000000000000, 1.836970198721030427E-16, -0.000000000000000000 ) ) ;
#3699=DIRECTION ( 'NONE',  ( -1.000000000000000000, 0.000000000000000000, 0.000000000000000000 ) ) ;
#3700=CARTESIAN_POINT ( 'NONE',  ( -601.1755229097230995, 36.95942061122438105, -15.32481103596387406 ) ) ;
#3706=CIRCLE ( 'NONE', #16456, 5.000000000000046185 ) ;
#3710=EDGE_CURVE ( 'NONE', #3578, #3746, #10435, .T. ) ;
#3725=CARTESIAN_POINT ( 'NONE',  ( -200.0000000000000000, -66.50000000000001421, 66.50000000000005684 ) ) ;
#3731=CARTESIAN_POINT ( 'NONE',  ( -211.2619052429883482, 0.000000000000000000, 0.000000000000000000 ) ) ;
#3738=DIRECTION ( 'NONE',  ( 0.000000000000000000, 0.000000000000000000, 1.000000000000000000 ) ) ;
#3739=FACE_BOUND ( 'NONE', #14612, .T. ) ;
#3745=DIRECTION ( 'NONE',  ( 0.000000000000000000, 0.000000000000000000, -1.000000000000000000 ) ) ;
#3746=VERTEX_POINT ( 'NONE', #11987 ) ;
#3754=ORIENTED_EDGE ( 'NONE', *, *, #8329, .T. ) ;
#3781=EDGE_CURVE ( 'NONE', #1564, #16348, #23216, .T. ) ;
#3782=EDGE_CURVE ( 'NONE', #23489, #14320, #20718, .T. ) ;
#3800=PRODUCT ( 'Pump housing', 'Pump housing', '', ( #2118 ) ) ;
#3801=CARTESIAN_POINT ( 'NONE',  ( -626.9846540392142060, 75.00000000000000000, 0.000000000000000000 ) ) ;
#3813=DIRECTION ( 'NONE',  ( 1.000000000000000000, 1.836970198721030427E-16, -0.000000000000000000 ) ) ;
#3815=AXIS2_PLACEMENT_3D ( 'NONE', #10264, #153, #12651 ) ;
#3828=VECTOR ( 'NONE', #6939, 1000.000000000000000 ) ;
#3837=CARTESIAN_POINT ( 'NONE',  ( -210.0000000000000284, 52.49999999999987210, 82.49999999999998579 ) ) ;
#3848=CARTESIAN_POINT ( 'NONE',  ( -200.0000000000000000, 52.50000000000007816, -52.49999999999999289 ) ) ;
#3859=ORIENTED_EDGE ( 'NONE', *, *, #17434, .F. ) ;
#3878=CARTESIAN_POINT ( 'NONE',  ( -626.9846540392142060, 75.00000000000000000, 74.99999999999991473 ) ) ;
#3880=LINE ( 'NONE', #11980, #5565 ) ;
#3904=ORIENTED_EDGE ( 'NONE', *, *, #8481, .F. ) ;
#3909=CARTESIAN_POINT ( 'NONE',  ( -726.9846540392142060, 66.50000000000009948, 71.50000000000005684 ) ) ;
#3911=CARTESIAN_POINT ( 'NONE',  ( -678.9461782662772293, 75.00000000000000000, 30.00000000000158096 ) ) ;
#3963=ADVANCED_FACE ( 'NONE', ( #3410 ), #25771, .F. ) ;
#3969=EDGE_CURVE ( 'NONE', #17794, #23789, #17238, .T. ) ;
#3987=DIRECTION ( 'NONE',  ( 0.000000000000000000, 1.000000000000000000, 0.000000000000000000 ) ) ;
#3988=SHAPE_DEFINITION_REPRESENTATION ( #20156, #24774 ) ;
#3996=ORIENTED_EDGE ( 'NONE', *, *, #20398, .F. ) ;
#4009=CARTESIAN_POINT ( 'NONE',  ( -210.0000000000000284, -82.49999999999990052, 52.49999999999977263 ) ) ;
#4014=DIRECTION ( 'NONE',  ( 0.000000000000000000, 0.000000000000000000, -1.000000000000000000 ) ) ;
#4023=DIRECTION ( 'NONE',  ( 0.000000000000000000, 1.000000000000000000, 0.000000000000000000 ) ) ;
#4030=ORIENTED_EDGE ( 'NONE', *, *, #25360, .F. ) ;
#4032=DIRECTION ( 'NONE',  ( 0.000000000000000000, 0.000000000000000000, 1.000000000000000000 ) ) ;
#4034=ORIENTED_EDGE ( 'NONE', *, *, #19887, .F. ) ;
#4052=CARTESIAN_POINT ( 'NONE',  ( -210.0000000000000284, -1.836970198721030378E-15, 0.000000000000000000 ) ) ;
#4093=DIRECTION ( 'NONE',  ( 0.000000000000000000, 0.000000000000000000, 1.000000000000000000 ) ) ;
#4106=EDGE_CURVE ( 'NONE', #9701, #3571, #21500, .T. ) ;
#4114=EDGE_CURVE ( 'NONE', #5117, #21778, #22040, .T. ) ;
#4120=EDGE_CURVE ( 'NONE', #15268, #9701, #13640, .T. ) ;
#4127=ORIENTED_EDGE ( 'NONE', *, *, #7691, .T. ) ;
#4153=CARTESIAN_POINT ( 'NONE',  ( -716.9846540392142060, 66.50000000000009948, -71.50000000000005684 ) ) ;
#4159=CARTESIAN_POINT ( 'NONE',  ( -726.9846540392142060, 0.000000000000000000, 0.000000000000000000 ) ) ;
#4173=EDGE_LOOP ( 'NONE', ( #25851, #18747, #17266, #5978 ) ) ;
#4181=CARTESIAN_POINT ( 'NONE',  ( -642.1644459338755269, 30.49398659613246920, 25.89371287723436055 ) ) ;
#4206=EDGE_CURVE ( 'NONE', #1180, #25953, #22281, .T. ) ;
#4208=CARTESIAN_POINT ( 'NONE',  ( -200.0000000000000000, 66.50000000000009948, -66.50000000000005684 ) ) ;
#4214=CARTESIAN_POINT ( 'NONE',  ( -210.0000000000000284, 71.50000000000009948, 66.50000000000005684 ) ) ;
#4219=ADVANCED_FACE ( 'NONE', ( #20279 ), #24134, .T. ) ;
#4263=EDGE_CURVE ( 'NONE', #9693, #1336, #13824, .T. ) ;
#4295=LINE ( 'NONE', #13845, #14879 ) ;
#4296=FACE_BOUND ( 'NONE', #23610, .T. ) ;
#4298=VERTEX_POINT ( 'NONE', #10298 ) ;
#4305=EDGE_CURVE ( 'NONE', #20514, #7340, #18405, .T. ) ;
#4315=CARTESIAN_POINT ( 'NONE',  ( -649.7157619631484522, 34.88051882544941407, 19.58372711145630518 ) ) ;
#4332=ORIENTED_EDGE ( 'NONE', *, *, #880, .T. ) ;
#4333=EDGE_LOOP ( 'NONE', ( #14082, #26052, #5291, #11582 ) ) ;
#4337=DIRECTION ( 'NONE',  ( -1.000000000000000000, 0.000000000000000000, 0.000000000000000000 ) ) ;
#4339=CARTESIAN_POINT ( 'NONE',  ( -716.9846540392142060, -66.50000000000001421, 71.50000000000005684 ) ) ;
#4354=AXIS2_PLACEMENT_3D ( 'NONE', #5482, #11211, #21208 ) ;
#4366=EDGE_CURVE ( 'NONE', #18580, #16641, #9577, .T. ) ;
#4390=ORIENTED_EDGE ( 'NONE', *, *, #25827, .T. ) ;
#4412=DIRECTION ( 'NONE',  ( 0.000000000000000000, 1.000000000000000000, 0.000000000000000000 ) ) ;
#4423=ORIENTED_EDGE ( 'NONE', *, *, #23315, .T. ) ;
#4427=ORIENTED_EDGE ( 'NONE', *, *, #5571, .F. ) ;
#4431=DIRECTION ( 'NONE',  ( 0.000000000000000000, 1.000000000000000000, 0.000000000000000000 ) ) ;
#4435=CARTESIAN_POINT ( 'NONE',  ( -626.9846540392142060, 95.00000000000000000, 0.000000000000000000 ) ) ;
#4438=CARTESIAN_POINT ( 'NONE',  ( -656.2662938234084322, 39.46402985900065374, 6.545868711047839739 ) ) ;
#4453=CARTESIAN_POINT ( 'NONE',  ( -598.8194166445492783, 39.91519017297324723, -20.78534762901812272 ) ) ;
#4458=CARTESIAN_POINT ( 'NONE',  ( -200.0000000000000000, 66.50000000000009948, 66.50000000000005684 ) ) ;
#4460=VERTEX_POINT ( 'NONE', #4464 ) ;
#4464=CARTESIAN_POINT ( 'NONE',  ( -626.9846540392142060, 75.00000000000000000, 74.99999999999991473 ) ) ;
#4466=DIRECTION ( 'NONE',  ( -1.000000000000000000, -1.836970198721030181E-16, 0.000000000000000000 ) ) ;
#4490=DIRECTION ( 'NONE',  ( -1.000000000000000000, 0.000000000000000000, 0.000000000000000000 ) ) ;
#4496=FACE_OUTER_BOUND ( 'NONE', #3080, .T. ) ;
#4513=VERTEX_POINT ( 'NONE', #12558 ) ;
#4516=AXIS2_PLACEMENT_3D ( 'NONE', #7888, #18267, #14015 ) ;
#4519=AXIS2_PLACEMENT_3D ( 'NONE', #17420, #19548, #17545 ) ;
#4526=EDGE_LOOP ( 'NONE', ( #6023, #12931 ) ) ;
#4533=AXIS2_PLACEMENT_3D ( 'NONE', #3557, #11401, #19524 ) ;
#4565=EDGE_LOOP ( 'NONE', ( #8568, #7532 ) ) ;
#4582=DIRECTION ( 'NONE',  ( 0.000000000000000000, 0.000000000000000000, 1.000000000000000000 ) ) ;
#4584=DIRECTION ( 'NONE',  ( 0.000000000000000000, 1.000000000000000000, 0.000000000000000000 ) ) ;
#4588=CARTESIAN_POINT ( 'NONE',  ( -615.3980966596806184, 30.54813962807670435, -33.04656978373367338 ) ) ;
#4589=ORIENTED_EDGE ( 'NONE', *, *, #12576, .F. ) ;
#4592=DIRECTION ( 'NONE',  ( 0.000000000000000000, 0.000000000000000000, 1.000000000000000000 ) ) ;
#4608=FACE_OUTER_BOUND ( 'NONE', #5489, .T. ) ;
#4634=AXIS2_PLACEMENT_3D ( 'NONE', #19307, #15685, #23560 ) ;
#4677=CARTESIAN_POINT ( 'NONE',  ( -716.9846540392142060, -52.49999999999972999, -82.49999999999998579 ) ) ;
#4684=CIRCLE ( 'NONE', #3390, 5.000000000000004441 ) ;
#4708=CARTESIAN_POINT ( 'NONE',  ( -652.7959024289831405, 36.96089747262086433, 15.32130098737787627 ) ) ;
#4715=CARTESIAN_POINT ( 'NONE',  ( -575.0231298121445889, 75.00000000000000000, 34.99999999999821654 ) ) ;
#4717=CARTESIAN_POINT ( 'NONE',  ( -659.9578749576080554, 43.44209025057394058, 11.75201215860449366 ) ) ;
#4724=CARTESIAN_POINT ( 'NONE',  ( -626.9846540392142060, 95.00000000000000000, 0.000000000000000000 ) ) ;
#4735=VECTOR ( 'NONE', #4757, 1000.000000000000000 ) ;
#4739=AXIS2_PLACEMENT_3D ( 'NONE', #23683, #7444, #10979 ) ;
#4749=DIRECTION ( 'NONE',  ( 0.000000000000000000, 1.000000000000000000, 0.000000000000000000 ) ) ;
#4752=VERTEX_POINT ( 'NONE', #3337 ) ;
#4757=DIRECTION ( 'NONE',  ( 1.000000000000000000, -0.000000000000000000, -0.000000000000000000 ) ) ;
#4766=DIRECTION ( 'NONE',  ( 0.000000000000000000, 0.000000000000000000, 1.000000000000000000 ) ) ;
#4772=AXIS2_PLACEMENT_3D ( 'NONE', #23209, #462, #4592 ) ;
#4779=EDGE_CURVE ( 'NONE', #2862, #21778, #11497, .T. ) ;
#4780=CARTESIAN_POINT ( 'NONE',  ( -200.0000000000000000, 0.000000000000000000, 0.000000000000000000 ) ) ;
#4782=EDGE_CURVE ( 'NONE', #4460, #8935, #23839, .T. ) ;
#4789=EDGE_CURVE ( 'NONE', #22711, #9566, #13628, .T. ) ;
#4795=AXIS2_PLACEMENT_3D ( 'NONE', #22185, #22049, #4093 ) ;
#4803=DIRECTION ( 'NONE',  ( 0.000000000000000000, 0.000000000000000000, 1.000000000000000000 ) ) ;
#4806=CARTESIAN_POINT ( 'NONE',  ( -626.9846540392140923, 26.45751311064577749, 30.00000000000005329 ) ) ;
#4813=FACE_BOUND ( 'NONE', #7599, .T. ) ;
#4814=DIRECTION ( 'NONE',  ( 0.000000000000000000, 1.000000000000000000, 0.000000000000000000 ) ) ;
#4834=LINE ( 'NONE', #4965, #14695 ) ;
#4843=DIRECTION ( 'NONE',  ( 1.000000000000000000, -0.000000000000000000, -0.000000000000000000 ) ) ;
#4847=CARTESIAN_POINT ( 'NONE',  ( -661.9833597215726968, 44.99899330872307246, 1.238957774783474797 ) ) ;
#4852=CARTESIAN_POINT ( 'NONE',  ( -614.3390598189121192, 30.96862867965382904, -32.65476733775240348 ) ) ;
#4855=DIRECTION ( 'NONE',  ( 0.000000000000000000, 0.000000000000000000, 1.000000000000000000 ) ) ;
#4859=ORIENTED_EDGE ( 'NONE', *, *, #8837, .F. ) ;
#4862=CARTESIAN_POINT ( 'NONE',  ( -716.9846540392142060, 52.49999999999986500, 82.49999999999998579 ) ) ;
#4875=ADVANCED_FACE ( 'NONE', ( #8507 ), #16185, .F. ) ;
#4894=CARTESIAN_POINT ( 'NONE',  ( -626.9846540392142060, 105.0000000000000000, -46.18033988749894547 ) ) ;
#4906=CARTESIAN_POINT ( 'NONE',  ( -575.0231298121445889, 90.00000000000000000, 34.99999999999821654 ) ) ;
#4909=ORIENTED_EDGE ( 'NONE', *, *, #18736, .F. ) ;
#4914=EDGE_LOOP ( 'NONE', ( #22151, #2094 ) ) ;
#4922=AXIS2_PLACEMENT_3D ( 'NONE', #7360, #19350, #19866 ) ;
#4930=CARTESIAN_POINT ( 'NONE',  ( -613.5337413356613752, 29.67126750635895149, 26.83244280794799153 ) ) ;
#4937=AXIS2_PLACEMENT_3D ( 'NONE', #18995, #2499, #11135 ) ;
#4941=CYLINDRICAL_SURFACE ( 'NONE', #11428, 5.000000000000004441 ) ;
#4950=CARTESIAN_POINT ( 'NONE',  ( -726.9846540392142060, -66.50000000000001421, 66.50000000000005684 ) ) ;
#4952=EDGE_LOOP ( 'NONE', ( #16647, #11731, #22184, #11956 ) ) ;
#4957=EDGE_LOOP ( 'NONE', ( #12266, #4589, #12791, #9802 ) ) ;
#4965=CARTESIAN_POINT ( 'NONE',  ( -716.9846540392142060, 52.49999999999991473, -82.49999999999998579 ) ) ;
#4981=DIRECTION ( 'NONE',  ( 0.000000000000000000, -1.000000000000000000, 0.000000000000000000 ) ) ;
#4985=AXIS2_PLACEMENT_3D ( 'NONE', #14141, #11740, #24261 ) ;
#4986=CARTESIAN_POINT ( 'NONE',  ( -601.6309025357880955, 37.98336425937555560, 24.13488029792940637 ) ) ;
#4987=EDGE_LOOP ( 'NONE', ( #4034, #1852, #15513, #10536 ) ) ;
#4991=ORIENTED_EDGE ( 'NONE', *, *, #22077, .F. ) ;
#4997=CARTESIAN_POINT ( 'NONE',  ( -575.0231298121466352, 90.00000000000000000, -30.00000000000202505 ) ) ;
#5000=DIRECTION ( 'NONE',  ( -1.000000000000000000, 0.000000000000000000, 0.000000000000000000 ) ) ;
#5014=ORIENTED_EDGE ( 'NONE', *, *, #687, .T. ) ;
#5017=EDGE_CURVE ( 'NONE', #3113, #5353, #13865, .T. ) ;
#5020=DIRECTION ( 'NONE',  ( 0.000000000000000000, 0.000000000000000000, 1.000000000000000000 ) ) ;
#5022=LINE ( 'NONE', #2765, #8306 ) ;
#5025=ADVANCED_FACE ( 'NONE', ( #18122 ), #1777, .F. ) ;
#5046=ORIENTED_EDGE ( 'NONE', *, *, #4366, .F. ) ;
#5052=DIRECTION ( 'NONE',  ( 0.000000000000000000, 0.000000000000000000, -1.000000000000000000 ) ) ;
#5060=DIRECTION ( 'NONE',  ( -1.000000000000000000, 0.000000000000000000, 0.000000000000000000 ) ) ;
#5098=CARTESIAN_POINT ( 'NONE',  ( -200.0000000000000000, -71.50000000000002842, -66.50000000000005684 ) ) ;
#5099=CARTESIAN_POINT ( 'NONE',  ( -716.9846540392142060, 52.50000000000007816, -52.49999999999999289 ) ) ;
#5100=AXIS2_PLACEMENT_3D ( 'NONE', #22642, #8795, #2546 ) ;
#5105=CARTESIAN_POINT ( 'NONE',  ( -626.9846540392142060, 28.28427124746186294, -34.99999999999999289 ) ) ;
#5110=EDGE_CURVE ( 'NONE', #10128, #2915, #19778, .T. ) ;
#5117=VERTEX_POINT ( 'NONE', #19250 ) ;
#5121=EDGE_CURVE ( 'NONE', #2152, #25083, #18521, .T. ) ;
#5151=CARTESIAN_POINT ( 'NONE',  ( -651.1759909824590977, 35.84781451397984853, -17.76753621510863468 ) ) ;
#5162=FACE_OUTER_BOUND ( 'NONE', #11393, .T. ) ;
#5163=CARTESIAN_POINT ( 'NONE',  ( -726.9846540392142060, 0.000000000000000000, 0.000000000000000000 ) ) ;
#5173=EDGE_LOOP ( 'NONE', ( #4427, #16912, #8399, #22391 ) ) ;
#5185=DIRECTION ( 'NONE',  ( 1.000000000000000000, 1.836970198721030427E-16, -0.000000000000000000 ) ) ;
#5194=ORIENTED_EDGE ( 'NONE', *, *, #15462, .T. ) ;
#5204=DIRECTION ( 'NONE',  ( 0.000000000000000000, 0.000000000000000000, 1.000000000000000000 ) ) ;
#5213=FACE_OUTER_BOUND ( 'NONE', #5173, .T. ) ;
#5237=ORIENTED_EDGE ( 'NONE', *, *, #15083, .T. ) ;
#5291=ORIENTED_EDGE ( 'NONE', *, *, #15160, .T. ) ;
#5295=DIRECTION ( 'NONE',  ( 1.000000000000000000, -0.000000000000000000, -0.000000000000000000 ) ) ;
#5297=DIRECTION ( 'NONE',  ( 0.000000000000000000, 0.000000000000000000, 1.000000000000000000 ) ) ;
#5317=AXIS2_PLACEMENT_3D ( 'NONE', #6691, #4584, #21071 ) ;
#5320=CARTESIAN_POINT ( 'NONE',  ( -200.0000000000000000, 61.50000000000009948, 66.50000000000005684 ) ) ;
#5328=ADVANCED_FACE ( 'NONE', ( #7083 ), #23323, .T. ) ;
#5343=EDGE_CURVE ( 'NONE', #4460, #2152, #13706, .T. ) ;
#5348=AXIS2_PLACEMENT_3D ( 'NONE', #68, #12298, #4337 ) ;
#5349=VECTOR ( 'NONE', #22440, 1000.000000000000000 ) ;
#5351=DIRECTION ( 'NONE',  ( 1.000000000000000000, -0.000000000000000000, -0.000000000000000000 ) ) ;
#5353=VERTEX_POINT ( 'NONE', #11708 ) ;
#5357=ORIENTED_EDGE ( 'NONE', *, *, #5017, .T. ) ;
#5361=CIRCLE ( 'NONE', #25392, 44.99999999999997158 ) ;
#5385=DIRECTION ( 'NONE',  ( 0.000000000000000000, 0.000000000000000000, 1.000000000000000000 ) ) ;
#5393=EDGE_CURVE ( 'NONE', #7095, #4298, #9853, .T. ) ;
#5394=CIRCLE ( 'NONE', #25792, 5.000000000000011546 ) ;
#5436=CARTESIAN_POINT ( 'NONE',  ( -616.1376504080243421, 28.58319296853060720, -27.98701491627070581 ) ) ;
#5452=CYLINDRICAL_SURFACE ( 'NONE', #4519, 5.000000000000095035 ) ;
#5456=ORIENTED_EDGE ( 'NONE', *, *, #19531, .F. ) ;
#5482=CARTESIAN_POINT ( 'NONE',  ( -626.9846540392142060, 75.00000000000000000, 0.000000000000000000 ) ) ;
#5483=CARTESIAN_POINT ( 'NONE',  ( -622.1697599706657229, 28.66687854691249981, 34.68786982843303690 ) ) ;
#5487=CARTESIAN_POINT ( 'NONE',  ( -726.9846540392142060, 66.50000000000009948, 66.50000000000005684 ) ) ;
#5489=EDGE_LOOP ( 'NONE', ( #22288, #9933, #13800, #10941 ) ) ;
#5527=AXIS2_PLACEMENT_3D ( 'NONE', #15478, #13360, #17734 ) ;
#5534=CARTESIAN_POINT ( 'NONE',  ( -211.2619052429883482, 0.000000000000000000, -75.00000000000000000 ) ) ;
#5541=EDGE_LOOP ( 'NONE', ( #2625, #9743, #15449, #16581 ) ) ;
#5546=ORIENTED_EDGE ( 'NONE', *, *, #1431, .F. ) ;
#5556=ADVANCED_FACE ( 'NONE', ( #19962, #24088, #13968, #2143, #12112, #18221, #10254, #24364 ), #22103, .T. ) ;
#5559=VECTOR ( 'NONE', #14133, 1000.000000000000000 ) ;
#5561=CARTESIAN_POINT ( 'NONE',  ( -614.3679688017556373, 29.30921813701808176, -27.22223345538390404 ) ) ;
#5562=EDGE_CURVE ( 'NONE', #15457, #16014, #295, .T. ) ;
#5565=VECTOR ( 'NONE', #20104, 1000.000000000000000 ) ;
#5571=EDGE_CURVE ( 'NONE', #7340, #1564, #11979, .T. ) ;
#5573=CARTESIAN_POINT ( 'NONE',  ( -200.0000000000000000, 69.99999999999998579, 0.000000000000000000 ) ) ;
#5576=VERTEX_POINT ( 'NONE', #16097 ) ;
#5577=ORIENTED_EDGE ( 'NONE', *, *, #4779, .T. ) ;
#5586=CARTESIAN_POINT ( 'NONE',  ( -265.6482238768269326, 4.898587196589409082E-15, 39.99999999999997158 ) ) ;
#5599=DIRECTION ( 'NONE',  ( 0.000000000000000000, 1.000000000000000000, 0.000000000000000000 ) ) ;
#5611=CARTESIAN_POINT ( 'NONE',  ( -716.9846540392142060, 52.50000000000007816, 52.49999999999999289 ) ) ;
#5631=DIRECTION ( 'NONE',  ( 1.000000000000000000, 1.836970198721030427E-16, -0.000000000000000000 ) ) ;
#5663=DIRECTION ( 'NONE',  ( -1.000000000000000000, -1.836970198721030181E-16, 0.000000000000000000 ) ) ;
#5675=VERTEX_POINT ( 'NONE', #22763 ) ;
#5679=AXIS2_PLACEMENT_3D ( 'NONE', #3653, #11760, #17871 ) ;
#5688=CARTESIAN_POINT ( 'NONE',  ( -600.2384622940975305, 37.62094780669912097, -13.59727104935886821 ) ) ;
#5704=ORIENTED_EDGE ( 'NONE', *, *, #5562, .T. ) ;
#5721=DIRECTION ( 'NONE',  ( 0.000000000000000000, 0.000000000000000000, 1.000000000000000000 ) ) ;
#5727=CARTESIAN_POINT ( 'NONE',  ( -626.9846540392142060, 90.00000000000000000, 0.000000000000000000 ) ) ;
#5754=EDGE_CURVE ( 'NONE', #19908, #16682, #24077, .T. ) ;
#5764=DIRECTION ( 'NONE',  ( 0.000000000000000000, -1.000000000000000000, 0.000000000000000000 ) ) ;
#5780=AXIS2_PLACEMENT_3D ( 'NONE', #23440, #21567, #713 ) ;
#5809=AXIS2_PLACEMENT_3D ( 'NONE', #11605, #1386, #1515 ) ;
#5813=ORIENTED_EDGE ( 'NONE', *, *, #15793, .T. ) ;
#5822=CARTESIAN_POINT ( 'NONE',  ( -716.9846540392142060, 52.49999999999991473, -82.49999999999998579 ) ) ;
#5827=DIRECTION ( 'NONE',  ( 0.000000000000000000, 0.000000000000000000, 1.000000000000000000 ) ) ;
#5835=EDGE_LOOP ( 'NONE', ( #16879, #24612, #16683, #7471, #4991 ) ) ;
#5858=FACE_BOUND ( 'NONE', #21745, .T. ) ;
#5863=ADVANCED_FACE ( 'NONE', ( #8596 ), #8726, .F. ) ;
#5873=FACE_OUTER_BOUND ( 'NONE', #18229, .T. ) ;
#5885=VERTEX_POINT ( 'NONE', #18976 ) ;
#5890=VECTOR ( 'NONE', #24298, 1000.000000000000000 ) ;
#5894=CARTESIAN_POINT ( 'NONE',  ( -636.9184764937167529, 28.24694889380673501, -28.32469577109011283 ) ) ;
#5900=EDGE_CURVE ( 'NONE', #2387, #11822, #25107, .T. ) ;
#5901=CYLINDRICAL_SURFACE ( 'NONE', #2947, 5.000000000000004441 ) ;
#5910=EDGE_CURVE ( 'NONE', #9153, #5885, #12571, .T. ) ;
#5917=CIRCLE ( 'NONE', #19504, 5.000000000000004441 ) ;
#5925=CARTESIAN_POINT ( 'NONE',  ( -200.0000000000000000, 61.50000000000009237, -66.50000000000005684 ) ) ;
#5955=CARTESIAN_POINT ( 'NONE',  ( -200.0000000000000000, -61.50000000000001421, 66.50000000000005684 ) ) ;
#5974=ORIENTED_EDGE ( 'NONE', *, *, #2171, .T. ) ;
#5978=ORIENTED_EDGE ( 'NONE', *, *, #26177, .T. ) ;
#5981=ORIENTED_EDGE ( 'NONE', *, *, #18822, .T. ) ;
#5984=DIRECTION ( 'NONE',  ( 0.000000000000000000, 0.000000000000000000, 1.000000000000000000 ) ) ;
#5995=CIRCLE ( 'NONE', #20876, 34.99999999999999289 ) ;
#5998=FACE_BOUND ( 'NONE', #1825, .T. ) ;
#6003=DIRECTION ( 'NONE',  ( -1.000000000000000000, -1.836970198721030181E-16, 0.000000000000000000 ) ) ;
#6010=ORIENTED_EDGE ( 'NONE', *, *, #19720, .T. ) ;
#6015=DIRECTION ( 'NONE',  ( 0.8802361161597900274, 5.811389476877145599E-17, 0.4745359626076074422 ) ) ;
#6017=CIRCLE ( 'NONE', #20890, 30.00000000000005329 ) ;
#6019=DIRECTION ( 'NONE',  ( 1.000000000000000000, 1.836970198721030427E-16, -0.000000000000000000 ) ) ;
#6023=ORIENTED_EDGE ( 'NONE', *, *, #16147, .T. ) ;
#6030=DIRECTION ( 'NONE',  ( 0.000000000000000000, 0.000000000000000000, 1.000000000000000000 ) ) ;
#6053=AXIS2_PLACEMENT_3D ( 'NONE', #9181, #13298, #17294 ) ;
#6078=ORIENTED_EDGE ( 'NONE', *, *, #8472, .F. ) ;
#6102=ORIENTED_EDGE ( 'NONE', *, *, #24595, .T. ) ;
#6105=VERTEX_POINT ( 'NONE', #21846 ) ;
#6109=ORIENTED_EDGE ( 'NONE', *, *, #19079, .F. ) ;
#6112=VERTEX_POINT ( 'NONE', #21459 ) ;
#6129=CARTESIAN_POINT ( 'NONE',  ( -626.9846540392142060, 90.00000000000000000, 0.000000000000000000 ) ) ;
#6140=DIRECTION ( 'NONE',  ( 0.000000000000000000, 0.000000000000000000, 1.000000000000000000 ) ) ;
#6146=EDGE_CURVE ( 'NONE', #87, #21399, #1123, .T. ) ;
#6159=CARTESIAN_POINT ( 'NONE',  ( -653.7331453363653964, 37.62258392649753347, 13.59271614633608571 ) ) ;
#6165=CARTESIAN_POINT ( 'NONE',  ( -716.9846540392142060, -66.50000000000001421, 66.50000000000005684 ) ) ;
#6170=DIRECTION ( 'NONE',  ( -1.000000000000000000, 0.000000000000000000, 0.000000000000000000 ) ) ;
#6172=DIRECTION ( 'NONE',  ( 0.000000000000000000, 0.000000000000000000, 1.000000000000000000 ) ) ;
#6183=CARTESIAN_POINT ( 'NONE',  ( -626.9846540392142060, 75.00000000000000000, -34.99999999999999289 ) ) ;
#6186=VECTOR ( 'NONE', #21766, 1000.000000000000114 ) ;
#6204=ORIENTED_EDGE ( 'NONE', *, *, #21012, .F. ) ;
#6208=EDGE_CURVE ( 'NONE', #21682, #17794, #20647, .T. ) ;
#6273=ORIENTED_EDGE ( 'NONE', *, *, #11560, .F. ) ;
#6279=VERTEX_POINT ( 'NONE', #24780 ) ;
#6286=CARTESIAN_POINT ( 'NONE',  ( -635.0888434903920370, 27.60293145401818649, 28.95600705801621544 ) ) ;
#6294=DIRECTION ( 'NONE',  ( 0.000000000000000000, -1.000000000000000000, 0.000000000000000000 ) ) ;
#6339=CARTESIAN_POINT ( 'NONE',  ( -726.9846540392142060, -52.49999999999991473, 82.49999999999998579 ) ) ;
#6362=VERTEX_POINT ( 'NONE', #5320 ) ;
#6363=CARTESIAN_POINT ( 'NONE',  ( -575.0231298121445889, 90.00000000000000000, 24.99999999999828759 ) ) ;
#6366=ORIENTED_EDGE ( 'NONE', *, *, #5910, .T. ) ;
#6375=ADVANCED_FACE ( 'NONE', ( #3579 ), #5452, .F. ) ;
#6382=EDGE_CURVE ( 'NONE', #23789, #13093, #9313, .T. ) ;
#6390=CARTESIAN_POINT ( 'NONE',  ( -575.0231298121466352, 75.00000000000000000, -35.00000000000203926 ) ) ;
#6411=AXIS2_PLACEMENT_3D ( 'NONE', #24230, #12373, #144 ) ;
#6418=CARTESIAN_POINT ( 'NONE',  ( -651.2040234678420347, 35.86671673404443084, 17.72972231506208018 ) ) ;
#6425=PLANE ( 'NONE',  #12130 ) ;
#6427=CARTESIAN_POINT ( 'NONE',  ( -660.9877162221778235, 44.22876715792673963, 8.378995438794239803 ) ) ;
#6437=EDGE_LOOP ( 'NONE', ( #20552, #22778 ) ) ;
#6443=DIRECTION ( 'NONE',  ( 0.000000000000000000, 0.000000000000000000, 1.000000000000000000 ) ) ;
#6493=VERTEX_POINT ( 'NONE', #18737 ) ;
#6499=CARTESIAN_POINT ( 'NONE',  ( -726.9846540392142060, -52.49999999999992895, -52.49999999999999289 ) ) ;
#6500=CARTESIAN_POINT ( 'NONE',  ( -575.0231298121466352, 75.00000000000000000, -30.00000000000202505 ) ) ;
#6503=DIRECTION ( 'NONE',  ( -0.000000000000000000, -1.000000000000000000, -0.000000000000000000 ) ) ;
#6520=FACE_BOUND ( 'NONE', #11424, .T. ) ;
#6521=DIRECTION ( 'NONE',  ( 1.000000000000000000, 1.836970198721030427E-16, -0.000000000000000000 ) ) ;
#6564=LINE ( 'NONE', #14682, #13263 ) ;
#6572=CARTESIAN_POINT ( 'NONE',  ( -626.9846540392097722, 90.00000000000000000, 54.99999999999995737 ) ) ;
#6594=CIRCLE ( 'NONE', #21470, 5.000000000000011546 ) ;
#6609=CIRCLE ( 'NONE', #16820, 69.99999999999998579 ) ;
#6623=AXIS2_PLACEMENT_3D ( 'NONE', #16430, #10715, #472 ) ;
#6635=DIRECTION ( 'NONE',  ( -1.000000000000000000, -1.836970198721030181E-16, 0.000000000000000000 ) ) ;
#6645=CARTESIAN_POINT ( 'NONE',  ( -597.0972138806185967, 39.91563328523288590, 2.647040059433892978 ) ) ;
#6653=FACE_BOUND ( 'NONE', #16421, .T. ) ;
#6654=CYLINDRICAL_SURFACE ( 'NONE', #17239, 29.99999999999999645 ) ;
#6656=ORIENTED_EDGE ( 'NONE', *, *, #11169, .F. ) ;
#6661=DIRECTION ( 'NONE',  ( 0.000000000000000000, 0.000000000000000000, 1.000000000000000000 ) ) ;
#6669=AXIS2_PLACEMENT_3D ( 'NONE', #15860, #1652, #14147 ) ;
#6678=CARTESIAN_POINT ( 'NONE',  ( -575.0231298121466352, 75.00000000000000000, -25.00000000000201794 ) ) ;
#6681=CARTESIAN_POINT ( 'NONE',  ( -655.3024676147620085, 38.75379567404313974, 9.955511827537780079 ) ) ;
#6691=CARTESIAN_POINT ( 'NONE',  ( -626.9846540392142060, 95.00000000000000000, 0.000000000000000000 ) ) ;
#6696=CARTESIAN_POINT ( 'NONE',  ( -592.1138474530150688, 44.89957181662549601, -3.064942242840709152 ) ) ;
#6702=ORIENTED_EDGE ( 'NONE', *, *, #25837, .F. ) ;
#6704=DIRECTION ( 'NONE',  ( -1.000000000000000000, 0.000000000000000000, 0.000000000000000000 ) ) ;
#6710=EDGE_CURVE ( 'NONE', #16682, #19908, #14923, .T. ) ;
#6734=CARTESIAN_POINT ( 'NONE',  ( -726.9846540392142060, -66.50000000000001421, 71.50000000000005684 ) ) ;
#6759=ORIENTED_EDGE ( 'NONE', *, *, #24291, .T. ) ;
#6768=DIRECTION ( 'NONE',  ( 0.000000000000000000, 0.000000000000000000, 1.000000000000000000 ) ) ;
#6785=CARTESIAN_POINT ( 'NONE',  ( -626.9846540392097722, 90.00000000000000000, 65.00000000000002842 ) ) ;
#6786=FACE_BOUND ( 'NONE', #7595, .T. ) ;
#6792=DIRECTION ( 'NONE',  ( 0.000000000000000000, 0.000000000000000000, 1.000000000000000000 ) ) ;
#6809=EDGE_CURVE ( 'NONE', #2387, #1721, #17460, .T. ) ;
#6815=DIRECTION ( 'NONE',  ( 0.000000000000000000, -1.000000000000000000, 0.000000000000000000 ) ) ;
#6823=CARTESIAN_POINT ( 'NONE',  ( -629.4215712140579626, 28.28427124746185228, 34.99999999999999289 ) ) ;
#6860=EDGE_CURVE ( 'NONE', #17170, #17304, #5995, .T. ) ;
#6862=VECTOR ( 'NONE', #25820, 1000.000000000000114 ) ;
#6899=CARTESIAN_POINT ( 'NONE',  ( -200.0000000000000000, 0.000000000000000000, 0.000000000000000000 ) ) ;
#6909=CARTESIAN_POINT ( 'NONE',  ( -616.1677987530077871, 28.57178177696692245, 27.99862729771767889 ) ) ;
#6916=DIRECTION ( 'NONE',  ( 0.000000000000000000, 0.000000000000000000, 1.000000000000000000 ) ) ;
#6938=CYLINDRICAL_SURFACE ( 'NONE', #15983, 5.000000000000004441 ) ;
#6939=DIRECTION ( 'NONE',  ( -0.000000000000000000, 1.000000000000000000, -0.000000000000000000 ) ) ;
#6947=FACE_OUTER_BOUND ( 'NONE', #24785, .T. ) ;
#6951=CARTESIAN_POINT ( 'NONE',  ( -658.1673319222918508, 42.09494090835337232, 16.06443073066892779 ) ) ;
#6957=CARTESIAN_POINT ( 'NONE',  ( -592.2265799526504679, 44.81207692804512988, 4.151637030843666309 ) ) ;
#6964=VERTEX_POINT ( 'NONE', #24870 ) ;
#6969=EDGE_CURVE ( 'NONE', #1593, #18580, #1177, .T. ) ;
#6971=CARTESIAN_POINT ( 'NONE',  ( -716.9846540392142060, 66.50000000000009948, -61.50000000000004974 ) ) ;
#6974=DIRECTION ( 'NONE',  ( -1.000000000000000000, -1.836970198721030181E-16, 0.000000000000000000 ) ) ;
#7011=LINE ( 'NONE', #15000, #25065 ) ;
#7020=EDGE_LOOP ( 'NONE', ( #13224, #188 ) ) ;
#7041=CARTESIAN_POINT ( 'NONE',  ( -603.3751967744402691, 35.45693745050460421, 18.53366164513259307 ) ) ;
#7066=ORIENTED_EDGE ( 'NONE', *, *, #19964, .T. ) ;
#7072=DIRECTION ( 'NONE',  ( 0.000000000000000000, 0.000000000000000000, -1.000000000000000000 ) ) ;
#7083=FACE_OUTER_BOUND ( 'NONE', #2951, .T. ) ;
#7088=CARTESIAN_POINT ( 'NONE',  ( -658.1427801728231088, 42.08087261121841038, -15.95318208560120610 ) ) ;
#7095=VERTEX_POINT ( 'NONE', #13023 ) ;
#7132=CARTESIAN_POINT ( 'NONE',  ( -648.7286587598725873, 34.24530595729361693, -20.67420341552261931 ) ) ;
#7156=CONICAL_SURFACE ( 'NONE', #22042, 39.99999999999997158, 0.4944367829892074018 ) ;
#7162=FACE_OUTER_BOUND ( 'NONE', #19770, .T. ) ;
#7165=CARTESIAN_POINT ( 'NONE',  ( -601.1835555497099222, 36.94693614929742154, 15.42485920190372717 ) ) ;
#7211=DIRECTION ( 'NONE',  ( 0.000000000000000000, -1.000000000000000000, 0.000000000000000000 ) ) ;
#7214=DIRECTION ( 'NONE',  ( -0.000000000000000000, 1.000000000000000000, -0.000000000000000000 ) ) ;
#7220=VERTEX_POINT ( 'NONE', #13651 ) ;
#7251=AXIS2_PLACEMENT_3D ( 'NONE', #1746, #13970, #17957 ) ;
#7256=CARTESIAN_POINT ( 'NONE',  ( -655.8738625874835861, 39.17324258975333606, -8.150688919272367272 ) ) ;
#7270=AXIS2_PLACEMENT_3D ( 'NONE', #3848, #7553, #11952 ) ;
#7272=EDGE_LOOP ( 'NONE', ( #10006, #18636 ) ) ;
#7277=CYLINDRICAL_SURFACE ( 'NONE', #24286, 30.00000000000000711 ) ;
#7282=ADVANCED_FACE ( 'NONE', ( #13749 ), #21876, .F. ) ;
#7289=DIRECTION ( 'NONE',  ( 0.000000000000000000, 0.000000000000000000, 1.000000000000000000 ) ) ;
#7308=CARTESIAN_POINT ( 'NONE',  ( -210.0000000000000568, 82.50000000000008527, 52.49999999999980105 ) ) ;
#7313=CARTESIAN_POINT ( 'NONE',  ( -211.2619052429883482, 9.184850993605148733E-15, 75.00000000000000000 ) ) ;
#7333=CARTESIAN_POINT ( 'NONE',  ( -265.6482238768269326, 0.000000000000000000, 0.000000000000000000 ) ) ;
#7340=VERTEX_POINT ( 'NONE', #14877 ) ;
#7353=FACE_OUTER_BOUND ( 'NONE', #13469, .T. ) ;
#7357=EDGE_CURVE ( 'NONE', #10760, #7340, #11767, .T. ) ;
#7360=CARTESIAN_POINT ( 'NONE',  ( -626.9846540392097722, 75.00000000000000000, 59.99999999999999289 ) ) ;
#7362=B_SPLINE_CURVE_WITH_KNOTS ( 'NONE', 3,
 ( #10697, #6823, #10420, #18668, #8961, #20811, #14805, #22807, #851, #24671, #14941, #24805, #455, #14545, #17070, #12414, #2582, #25204, #8695, #18537, #6951, #20540, #16806, #4717, #12822, #2311, #6427, #20944, #22675, #319, #23076, #2722, #4847, #10827, #18942, #722, #15574, #25708, #13578, #17193, #17325, #11331, #19575, #7088, #21705, #25587, #23698, #13458, #17448, #19200, #21452, #15446, #15202, #2976, #23574, #9464, #25331, #1366, #3103, #21204, #19447, #23330, #15699, #5105 ),
 .UNSPECIFIED., .F., .F.,
 ( 4, 2, 2, 2, 2, 2, 2, 2, 2, 2, 2, 2, 2, 2, 2, 2, 2, 2, 2, 2, 2, 2, 2, 2, 2, 2, 2, 2, 2, 2, 2, 4 ),
 ( 0.1150183322533817887, 0.1222062663255236575, 0.1258002333615945989, 0.1293942003976655264, 0.1329881674337364816, 0.1365821344698074091, 0.1437700685419490421, 0.1455670520599845474, 0.1473640355780200806, 0.1509580026140910913, 0.1581459366862331684, 0.1599429202042686182, 0.1617399037223040681, 0.1653338707583749956, 0.1671308542764104454, 0.1689278377944458953, 0.1725218048305168228, 0.1761157718665877225, 0.1779127553846231724, 0.1797097389026586223, 0.1868976729748003107, 0.1886946564928357883, 0.1904916400108712105, 0.1940856070469419992, 0.1976795740830127324, 0.2012735411190835211, 0.2084614751912248487, 0.2120554422272953876, 0.2156494092633658988, 0.2192433762994364654, 0.2228373433355070321, 0.2300252774076481099 ),
 .UNSPECIFIED. ) ;
#7390=DIRECTION ( 'NONE',  ( -1.000000000000000000, 0.000000000000000000, 0.000000000000000000 ) ) ;
#7400=ORIENTED_EDGE ( 'NONE', *, *, #21432, .F. ) ;
#7410=CARTESIAN_POINT ( 'NONE',  ( -210.0000000000000284, 69.99999999999998579, 0.000000000000000000 ) ) ;
#7420=VERTEX_POINT ( 'NONE', #14610 ) ;
#7424=EDGE_CURVE ( 'NONE', #26265, #19296, #8498, .T. ) ;
#7437=VECTOR ( 'NONE', #8707, 1000.000000000000000 ) ;
#7444=DIRECTION ( 'NONE',  ( 0.000000000000000000, 1.000000000000000000, 0.000000000000000000 ) ) ;
#7445=CARTESIAN_POINT ( 'NONE',  ( -626.9846540392142060, 105.0000000000000000, 0.000000000000000000 ) ) ;
#7459=AXIS2_PLACEMENT_3D ( 'NONE', #16031, #26038, #24156 ) ;
#7464=CARTESIAN_POINT ( 'NONE',  ( -678.9461782662789346, 75.00000000000000000, -29.99999999999836220 ) ) ;
#7466=ORIENTED_EDGE ( 'NONE', *, *, #20455, .F. ) ;
#7471=ORIENTED_EDGE ( 'NONE', *, *, #12728, .T. ) ;
#7476=CIRCLE ( 'NONE', #1548, 5.000000000000046185 ) ;
#7481=CIRCLE ( 'NONE', #10910, 30.00000000000000000 ) ;
#7498=VERTEX_POINT ( 'NONE', #6363 ) ;
#7506=EDGE_CURVE ( 'NONE', #19428, #6493, #322, .T. ) ;
#7522=DIRECTION ( 'NONE',  ( -1.000000000000000000, 0.000000000000000000, 0.000000000000000000 ) ) ;
#7527=ORIENTED_EDGE ( 'NONE', *, *, #9629, .T. ) ;
#7532=ORIENTED_EDGE ( 'NONE', *, *, #9614, .F. ) ;
#7544=CARTESIAN_POINT ( 'NONE',  ( -605.2086264830600157, 34.26251070455288072, -20.65666574593837268 ) ) ;
#7550=CARTESIAN_POINT ( 'NONE',  ( -716.9846540392142060, 82.50000000000008527, -52.49999999999977973 ) ) ;
#7553=DIRECTION ( 'NONE',  ( -1.000000000000000000, -1.836970198721030181E-16, 0.000000000000000000 ) ) ;
#7560=CARTESIAN_POINT ( 'NONE',  ( -210.0000000000000284, 61.50000000000009948, 66.50000000000005684 ) ) ;
#7566=DIRECTION ( 'NONE',  ( 0.000000000000000000, 1.000000000000000000, 0.000000000000000000 ) ) ;
#7571=DIRECTION ( 'NONE',  ( 0.000000000000000000, 0.000000000000000000, -1.000000000000000000 ) ) ;
#7572=CARTESIAN_POINT ( 'NONE',  ( -678.9461782662772293, 90.00000000000000000, 30.00000000000158096 ) ) ;
#7589=ORIENTED_EDGE ( 'NONE', *, *, #13932, .F. ) ;
#7592=CARTESIAN_POINT ( 'NONE',  ( -624.5543896866091700, 28.38207856527901995, 34.92076931028241660 ) ) ;
#7595=EDGE_LOOP ( 'NONE', ( #15956, #1490 ) ) ;
#7599=EDGE_LOOP ( 'NONE', ( #3520, #20246 ) ) ;
#7613=FACE_OUTER_BOUND ( 'NONE', #25812, .T. ) ;
#7644=CARTESIAN_POINT ( 'NONE',  ( -716.9846540392142060, -66.50000000000001421, 66.50000000000005684 ) ) ;
#7651=VERTEX_POINT ( 'NONE', #23900 ) ;
#7661=CIRCLE ( 'NONE', #8109, 34.99999999999999289 ) ;
#7671=AXIS2_PLACEMENT_3D ( 'NONE', #7728, #15840, #4032 ) ;
#7687=ORIENTED_EDGE ( 'NONE', *, *, #25360, .T. ) ;
#7688=ORIENTED_EDGE ( 'NONE', *, *, #21906, .F. ) ;
#7691=EDGE_CURVE ( 'NONE', #13855, #15801, #3706, .T. ) ;
#7698=CARTESIAN_POINT ( 'NONE',  ( -210.0000000000000284, -66.50000000000001421, 66.50000000000005684 ) ) ;
#7716=AXIS2_PLACEMENT_3D ( 'NONE', #21336, #1493, #11335 ) ;
#7728=CARTESIAN_POINT ( 'NONE',  ( -716.9846540392142060, 66.50000000000009948, -66.50000000000005684 ) ) ;
#7731=ORIENTED_EDGE ( 'NONE', *, *, #18822, .F. ) ;
#7753=CARTESIAN_POINT ( 'NONE',  ( -210.0000000000000284, 71.50000000000009948, 66.50000000000005684 ) ) ;
#7758=ORIENTED_EDGE ( 'NONE', *, *, #8481, .T. ) ;
#7766=CARTESIAN_POINT ( 'NONE',  ( -575.0231298121466352, 75.00000000000000000, -30.00000000000202505 ) ) ;
#7796=EDGE_CURVE ( 'NONE', #14640, #11418, #23008, .T. ) ;
#7797=CARTESIAN_POINT ( 'NONE',  ( -716.9846540392142060, 82.50000000000008527, 52.49999999999980105 ) ) ;
#7810=ORIENTED_EDGE ( 'NONE', *, *, #15462, .F. ) ;
#7813=DIRECTION ( 'NONE',  ( 1.000000000000000000, -0.000000000000000000, -0.000000000000000000 ) ) ;
#7816=ORIENTED_EDGE ( 'NONE', *, *, #16318, .T. ) ;
#7828=EDGE_CURVE ( 'NONE', #8666, #26151, #17362, .T. ) ;
#7859=ORIENTED_EDGE ( 'NONE', *, *, #7506, .T. ) ;
#7874=CARTESIAN_POINT ( 'NONE',  ( -626.9846540392142060, 26.45751311064579880, -30.00000000000005329 ) ) ;
#7888=CARTESIAN_POINT ( 'NONE',  ( -716.9846540392142060, -52.49999999999991473, 82.49999999999998579 ) ) ;
#7950=VERTEX_POINT ( 'NONE', #17233 ) ;
#7953=CARTESIAN_POINT ( 'NONE',  ( -626.9846540392142060, 95.00000000000000000, 0.000000000000000000 ) ) ;
#7964=DIRECTION ( 'NONE',  ( 1.000000000000000000, 1.836970198721030427E-16, -0.000000000000000000 ) ) ;
#7987=VERTEX_POINT ( 'NONE', #6734 ) ;
#7989=CARTESIAN_POINT ( 'NONE',  ( -200.0000000000000000, 52.49999999999988631, -82.49999999999998579 ) ) ;
#7994=CARTESIAN_POINT ( 'NONE',  ( 0.000000000000000000, 0.000000000000000000, 0.000000000000000000 ) ) ;
#7995=CARTESIAN_POINT ( 'NONE',  ( -626.9846540392097722, 90.00000000000000000, 59.99999999999999289 ) ) ;
#8002=VERTEX_POINT ( 'NONE', #25373 ) ;
#8030=ORIENTED_EDGE ( 'NONE', *, *, #26271, .T. ) ;
#8064=ORIENTED_EDGE ( 'NONE', *, *, #10595, .T. ) ;
#8067=ADVANCED_FACE ( 'NONE', ( #20980 ), #10867, .T. ) ;
#8072=LINE ( 'NONE', #7797, #25352 ) ;
#8073=CARTESIAN_POINT ( 'NONE',  ( -726.9846540392142060, -52.49999999999972999, -82.49999999999998579 ) ) ;
#8090=ORIENTED_EDGE ( 'NONE', *, *, #5017, .F. ) ;
#8094=EDGE_LOOP ( 'NONE', ( #21217, #8700 ) ) ;
#8097=EDGE_CURVE ( 'NONE', #16256, #6362, #22153, .T. ) ;
#8107=VECTOR ( 'NONE', #1463, 1000.000000000000000 ) ;
#8109=AXIS2_PLACEMENT_3D ( 'NONE', #10823, #14936, #20940 ) ;
#8115=FACE_BOUND ( 'NONE', #9067, .T. ) ;
#8134=EDGE_LOOP ( 'NONE', ( #23670, #25437, #24038, #18738 ) ) ;
#8135=VECTOR ( 'NONE', #4431, 1000.000000000000000 ) ;
#8140=ORIENTED_EDGE ( 'NONE', *, *, #11404, .T. ) ;
#8149=CARTESIAN_POINT ( 'NONE',  ( -656.7826941990241494, 39.84779524062224709, 4.035097616097491624 ) ) ;
#8150=AXIS2_PLACEMENT_3D ( 'NONE', #2988, #19713, #13467 ) ;
#8159=DIRECTION ( 'NONE',  ( 0.000000000000000000, 0.000000000000000000, 1.000000000000000000 ) ) ;
#8170=EDGE_LOOP ( 'NONE', ( #2942, #2696, #18443, #20520 ) ) ;
#8223=ORIENTED_EDGE ( 'NONE', *, *, #22077, .T. ) ;
#8246=DIRECTION ( 'NONE',  ( 0.000000000000000000, 1.000000000000000000, 0.000000000000000000 ) ) ;
#8248=FACE_BOUND ( 'NONE', #8296, .T. ) ;
#8257=CYLINDRICAL_SURFACE ( 'NONE', #2548, 5.000000000000011546 ) ;
#8259=CARTESIAN_POINT ( 'NONE',  ( -200.0000000000000000, -82.49999999999990052, 52.49999999999977263 ) ) ;
#8260=SHAPE_REPRESENTATION_RELATIONSHIP ( 'NONE' , 'NONE' ,  #24774, #25803 ) ;
#8267=ORIENTED_EDGE ( 'NONE', *, *, #1200, .T. ) ;
#8285=FACE_OUTER_BOUND ( 'NONE', #12089, .T. ) ;
#8296=EDGE_LOOP ( 'NONE', ( #1202, #23202 ) ) ;
#8300=VECTOR ( 'NONE', #3378, 1000.000000000000000 ) ;
#8306=VECTOR ( 'NONE', #13372, 1000.000000000000000 ) ;
#8308=VECTOR ( 'NONE', #13906, 1000.000000000000000 ) ;
#8310=VECTOR ( 'NONE', #11872, 1000.000000000000000 ) ;
#8329=EDGE_CURVE ( 'NONE', #14785, #21989, #13496, .T. ) ;
#8339=AXIS2_PLACEMENT_3D ( 'NONE', #6500, #2520, #254 ) ;
#8388=ORIENTED_EDGE ( 'NONE', *, *, #532, .T. ) ;
#8394=EDGE_LOOP ( 'NONE', ( #18245, #13365, #24746, #17608 ) ) ;
#8399=ORIENTED_EDGE ( 'NONE', *, *, #869, .T. ) ;
#8411=CARTESIAN_POINT ( 'NONE',  ( -654.3715413940425378, 38.07917292905567308, 12.25576229706686426 ) ) ;
#8425=DIRECTION ( 'NONE',  ( -0.000000000000000000, -1.000000000000000000, -0.000000000000000000 ) ) ;
#8431=EDGE_LOOP ( 'NONE', ( #10734, #1503 ) ) ;
#8440=DIRECTION ( 'NONE',  ( 0.000000000000000000, -1.000000000000000000, 0.000000000000000000 ) ) ;
#8466=CARTESIAN_POINT ( 'NONE',  ( -626.9846540392097722, 75.00000000000000000, 59.99999999999999289 ) ) ;
#8472=EDGE_CURVE ( 'NONE', #10135, #6105, #3203, .T. ) ;
#8481=EDGE_CURVE ( 'NONE', #6964, #1593, #21068, .T. ) ;
#8498=LINE ( 'NONE', #658, #14322 ) ;
#8507=FACE_OUTER_BOUND ( 'NONE', #14079, .T. ) ;
#8510=PLANE ( 'NONE',  #18077 ) ;
#8548=CARTESIAN_POINT ( 'NONE',  ( -639.6132534865922707, 29.31434396970803036, 27.21671984979430547 ) ) ;
#8557=VECTOR ( 'NONE', #13308, 1000.000000000000000 ) ;
#8564=CARTESIAN_POINT ( 'NONE',  ( -608.4139831770295359, 33.82757453087469912, -29.68732721380340678 ) ) ;
#8568=ORIENTED_EDGE ( 'NONE', *, *, #22836, .F. ) ;
#8591=EDGE_CURVE ( 'NONE', #7950, #5117, #21347, .T. ) ;
#8596=FACE_OUTER_BOUND ( 'NONE', #1988, .T. ) ;
#8633=EDGE_CURVE ( 'NONE', #15830, #17701, #24958, .T. ) ;
#8652=DIRECTION ( 'NONE',  ( -1.000000000000000000, 0.000000000000000000, 0.000000000000000000 ) ) ;
#8657=FACE_OUTER_BOUND ( 'NONE', #24237, .T. ) ;
#8666=VERTEX_POINT ( 'NONE', #17340 ) ;
#8686=CARTESIAN_POINT ( 'NONE',  ( -656.1498148884619468, 39.37764844114641960, 7.046424841349725021 ) ) ;
#8695=CARTESIAN_POINT ( 'NONE',  ( -655.1625848890473662, 39.92241353143312921, 20.79055835074375480 ) ) ;
#8699=CARTESIAN_POINT ( 'NONE',  ( -601.6618123970941951, 37.95920655747095651, -24.18560810059053168 ) ) ;
#8700=ORIENTED_EDGE ( 'NONE', *, *, #19855, .F. ) ;
#8705=ORIENTED_EDGE ( 'NONE', *, *, #10544, .F. ) ;
#8707=DIRECTION ( 'NONE',  ( 1.000000000000000000, -0.000000000000000000, -0.000000000000000000 ) ) ;
#8726=CYLINDRICAL_SURFACE ( 'NONE', #11297, 5.000000000000046185 ) ;
#8741=CARTESIAN_POINT ( 'NONE',  ( -626.9846540392142060, 75.00000000000000000, -65.00000000000004263 ) ) ;
#8746=CARTESIAN_POINT ( 'NONE',  ( -210.0000000000000284, 52.49999999999988631, -82.49999999999998579 ) ) ;
#8769=AXIS2_PLACEMENT_3D ( 'NONE', #7995, #22252, #19494 ) ;
#8770=CARTESIAN_POINT ( 'NONE',  ( -726.9846540392142060, 82.50000000000008527, 52.49999999999980105 ) ) ;
#8789=DIRECTION ( 'NONE',  ( 0.000000000000000000, 0.000000000000000000, 1.000000000000000000 ) ) ;
#8792=ORIENTED_EDGE ( 'NONE', *, *, #3782, .T. ) ;
#8795=DIRECTION ( 'NONE',  ( 0.000000000000000000, 1.000000000000000000, 0.000000000000000000 ) ) ;
#8804=AXIS2_PLACEMENT_3D ( 'NONE', #19728, #6974, #13478 ) ;
#8805=ORIENTED_EDGE ( 'NONE', *, *, #6809, .F. ) ;
#8823=DIRECTION ( 'NONE',  ( 0.000000000000000000, 0.000000000000000000, -1.000000000000000000 ) ) ;
#8832=CARTESIAN_POINT ( 'NONE',  ( -599.4467069854360943, 39.47241407940956037, 21.63078978636851346 ) ) ;
#8837=EDGE_CURVE ( 'NONE', #6493, #11418, #11598, .T. ) ;
#8839=ORIENTED_EDGE ( 'NONE', *, *, #16631, .T. ) ;
#8840=ORIENTED_EDGE ( 'NONE', *, *, #25417, .T. ) ;
#8866=ORIENTED_EDGE ( 'NONE', *, *, #18736, .T. ) ;
#8888=DIRECTION ( 'NONE',  ( -1.000000000000000000, -1.836970198721030181E-16, 0.000000000000000000 ) ) ;
#8897=CARTESIAN_POINT ( 'NONE',  ( -210.0000000000000284, -66.50000000000001421, -66.50000000000005684 ) ) ;
#8901=AXIS2_PLACEMENT_3D ( 'NONE', #18734, #24734, #517 ) ;
#8910=CARTESIAN_POINT ( 'NONE',  ( -200.0000000000000000, 52.49999999999988631, -82.49999999999998579 ) ) ;
#8913=CARTESIAN_POINT ( 'NONE',  ( -611.0434898207377046, 30.88177058762790850, 25.43160472393209659 ) ) ;
#8929=CIRCLE ( 'NONE', #11870, 69.99999999999998579 ) ;
#8935=VERTEX_POINT ( 'NONE', #20657 ) ;
#8938=DIRECTION ( 'NONE',  ( 1.000000000000000000, -0.000000000000000000, -0.000000000000000000 ) ) ;
#8949=AXIS2_PLACEMENT_3D ( 'NONE', #4950, #16645, #6661 ) ;
#8961=CARTESIAN_POINT ( 'NONE',  ( -636.4062240200004226, 29.79465556942914972, 33.72744621685050959 ) ) ;
#8966=CARTESIAN_POINT ( 'NONE',  ( -619.3049992912841617, 29.30303271858384306, -34.15210011782420452 ) ) ;
#9001=CIRCLE ( 'NONE', #13249, 69.99999999999998579 ) ;
#9003=DIRECTION ( 'NONE',  ( 0.000000000000000000, -1.000000000000000000, 0.000000000000000000 ) ) ;
#9011=EDGE_CURVE ( 'NONE', #16736, #2387, #6609, .T. ) ;
#9012=DIRECTION ( 'NONE',  ( 1.000000000000000000, -0.000000000000000000, 1.224646799147353207E-16 ) ) ;
#9019=CIRCLE ( 'NONE', #23051, 5.000000000000004441 ) ;
#9025=DIRECTION ( 'NONE',  ( 1.000000000000000000, -0.000000000000000000, -0.000000000000000000 ) ) ;
#9033=EDGE_LOOP ( 'NONE', ( #1630, #21463, #8140, #18034 ) ) ;
#9067=EDGE_LOOP ( 'NONE', ( #17634, #5704 ) ) ;
#9073=CARTESIAN_POINT ( 'NONE',  ( -626.9846540392142060, 90.00000000000000000, -65.00000000000004263 ) ) ;
#9078=LINE ( 'NONE', #11197, #25365 ) ;
#9092=CARTESIAN_POINT ( 'NONE',  ( -622.1724833024856025, 28.60431887920636740, -34.74667818490387816 ) ) ;
#9118=ORIENTED_EDGE ( 'NONE', *, *, #7796, .F. ) ;
#9134=CARTESIAN_POINT ( 'NONE',  ( -626.9846540392142060, 90.00000000000000000, -34.99999999999999289 ) ) ;
#9153=VERTEX_POINT ( 'NONE', #8259 ) ;
#9161=AXIS2_PLACEMENT_3D ( 'NONE', #4159, #20110, #3745 ) ;
#9170=AXIS2_PLACEMENT_3D ( 'NONE', #7766, #22163, #13500 ) ;
#9176=AXIS2_PLACEMENT_3D ( 'NONE', #19103, #25622, #1398 ) ;
#9181=CARTESIAN_POINT ( 'NONE',  ( -210.0000000000000284, -66.50000000000001421, 66.50000000000005684 ) ) ;
#9204=VECTOR ( 'NONE', #3157, 1000.000000000000000 ) ;
#9210=DIRECTION ( 'NONE',  ( 0.000000000000000000, 0.000000000000000000, -1.000000000000000000 ) ) ;
#9215=DIRECTION ( 'NONE',  ( -1.000000000000000000, -1.836970198721030181E-16, 0.000000000000000000 ) ) ;
#9220=AXIS2_PLACEMENT_3D ( 'NONE', #5727, #143, #16364 ) ;
#9237=ADVANCED_FACE ( 'NONE', ( #12788, #20915, #2694, #10799, #4296, #12386 ), #18910, .F. ) ;
#9262=CARTESIAN_POINT ( 'NONE',  ( -654.8952864718139608, 38.45762375594820526, -11.01125294513469122 ) ) ;
#9287=ADVANCED_FACE ( 'NONE', ( #18419 ), #12173, .F. ) ;
#9298=CARTESIAN_POINT ( 'NONE',  ( -599.8048379379712287, 37.93045404823428868, -12.70834960012116710 ) ) ;
#9313=LINE ( 'NONE', #7308, #19368 ) ;
#9334=CIRCLE ( 'NONE', #3815, 44.99999999999997158 ) ;
#9344=CARTESIAN_POINT ( 'NONE',  ( -626.9846540392142060, -82.50099999999990530, 0.000000000000000000 ) ) ;
#9370=FACE_OUTER_BOUND ( 'NONE', #18612, .T. ) ;
#9376=ADVANCED_FACE ( 'NONE', ( #2204 ), #14297, .T. ) ;
#9401=VECTOR ( 'NONE', #18233, 1000.000000000000000 ) ;
#9416=DIRECTION ( 'NONE',  ( 1.000000000000000000, -0.000000000000000000, -0.000000000000000000 ) ) ;
#9419=CARTESIAN_POINT ( 'NONE',  ( -210.0000000000000284, 61.50000000000009237, -66.50000000000005684 ) ) ;
#9422=CARTESIAN_POINT ( 'NONE',  ( -619.8916681553856733, 27.37461815474928173, -29.16715517154350934 ) ) ;
#9437=ORIENTED_EDGE ( 'NONE', *, *, #3123, .T. ) ;
#9440=CARTESIAN_POINT ( 'NONE',  ( -210.0000000000000000, -82.49999999999991473, -52.49999999999977973 ) ) ;
#9441=ORIENTED_EDGE ( 'NONE', *, *, #880, .F. ) ;
#9464=CARTESIAN_POINT ( 'NONE',  ( -642.7011836544691050, 32.34672097386517464, -31.29233336928180620 ) ) ;
#9470=CARTESIAN_POINT ( 'NONE',  ( -612.2488540682973053, 31.87925413264133923, 31.76643078590619851 ) ) ;
#9476=ORIENTED_EDGE ( 'NONE', *, *, #4206, .F. ) ;
#9480=EDGE_CURVE ( 'NONE', #8002, #21682, #19361, .T. ) ;
#9502=VERTEX_POINT ( 'NONE', #6971 ) ;
#9521=CARTESIAN_POINT ( 'NONE',  ( -726.9846540392142060, 52.50000000000007816, -52.49999999999999289 ) ) ;
#9559=( GEOMETRIC_REPRESENTATION_CONTEXT ( 3 ) GLOBAL_UNCERTAINTY_ASSIGNED_CONTEXT ( ( #17337 ) ) GLOBAL_UNIT_ASSIGNED_CONTEXT ( ( #12387, #15836, #1895 ) ) REPRESENTATION_CONTEXT ( 'NONE', 'WORKASPACE' ) );
#9566=VERTEX_POINT ( 'NONE', #6572 ) ;
#9570=AXIS2_PLACEMENT_3D ( 'NONE', #18264, #16802, #24669 ) ;
#9577=CIRCLE ( 'NONE', #24468, 4.999999999999997335 ) ;
#9580=DIRECTION ( 'NONE',  ( 0.000000000000000000, 1.000000000000000000, 0.000000000000000000 ) ) ;
#9600=CARTESIAN_POINT ( 'NONE',  ( -626.3753644243258805, 28.28427124746188426, 34.99999999999999289 ) ) ;
#9609=ORIENTED_EDGE ( 'NONE', *, *, #23617, .F. ) ;
#9614=EDGE_CURVE ( 'NONE', #17336, #25302, #14688, .T. ) ;
#9615=LINE ( 'NONE', #15848, #11397 ) ;
#9624=CARTESIAN_POINT ( 'NONE',  ( -210.0000000000000284, 0.000000000000000000, 0.000000000000000000 ) ) ;
#9629=EDGE_CURVE ( 'NONE', #14320, #567, #2996, .T. ) ;
#9636=ORIENTED_EDGE ( 'NONE', *, *, #2842, .F. ) ;
#9639=VECTOR ( 'NONE', #4412, 1000.000000000000000 ) ;
#9675=FACE_OUTER_BOUND ( 'NONE', #24373, .T. ) ;
#9681=CARTESIAN_POINT ( 'NONE',  ( -597.1859489463258797, 39.84828722673089629, -4.032642683987440968 ) ) ;
#9689=DIRECTION ( 'NONE',  ( -1.000000000000000000, -1.836970198721030181E-16, 0.000000000000000000 ) ) ;
#9692=CARTESIAN_POINT ( 'NONE',  ( -210.0000000000000284, -66.50000000000001421, 66.50000000000005684 ) ) ;
#9693=VERTEX_POINT ( 'NONE', #25725 ) ;
#9700=CIRCLE ( 'NONE', #10148, 5.000000000000011546 ) ;
#9701=VERTEX_POINT ( 'NONE', #21466 ) ;
#9721=VECTOR ( 'NONE', #13108, 1000.000000000000000 ) ;
#9722=EDGE_CURVE ( 'NONE', #13093, #10307, #9615, .T. ) ;
#9743=ORIENTED_EDGE ( 'NONE', *, *, #21185, .F. ) ;
#9770=EDGE_CURVE ( 'NONE', #15457, #18983, #23845, .T. ) ;
#9796=EDGE_LOOP ( 'NONE', ( #6702, #20609, #2588, #6109, #20081, #18332, #1767, #2123 ) ) ;
#9802=ORIENTED_EDGE ( 'NONE', *, *, #8633, .T. ) ;
#9815=VECTOR ( 'NONE', #20521, 1000.000000000000000 ) ;
#9829=ORIENTED_EDGE ( 'NONE', *, *, #3363, .T. ) ;
#9830=ORIENTED_EDGE ( 'NONE', *, *, #3710, .T. ) ;
#9839=FACE_OUTER_BOUND ( 'NONE', #9033, .T. ) ;
#9853=LINE ( 'NONE', #16236, #13439 ) ;
#9858=CIRCLE ( 'NONE', #21348, 5.000000000000004441 ) ;
#9869=EDGE_LOOP ( 'NONE', ( #14516, #18953, #16851, #21083 ) ) ;
#9883=CARTESIAN_POINT ( 'NONE',  ( -629.5673161569764034, 26.57848330823986771, -29.89298347762988328 ) ) ;
#9907=DIRECTION ( 'NONE',  ( 0.000000000000000000, -1.000000000000000000, 0.000000000000000000 ) ) ;
#9909=DIRECTION ( 'NONE',  ( 0.000000000000000000, 0.000000000000000000, 1.000000000000000000 ) ) ;
#9931=CARTESIAN_POINT ( 'NONE',  ( -716.9846540392142060, -52.49999999999991473, 82.49999999999998579 ) ) ;
#9933=ORIENTED_EDGE ( 'NONE', *, *, #21432, .T. ) ;
#9939=LINE ( 'NONE', #22061, #13436 ) ;
#9946=ADVANCED_FACE ( 'NONE', ( #14135, #13998 ), #22129, .T. ) ;
#9962=VERTEX_POINT ( 'NONE', #3909 ) ;
#9971=DIRECTION ( 'NONE',  ( 0.000000000000000000, -1.000000000000000000, 0.000000000000000000 ) ) ;
#10001=ORIENTED_EDGE ( 'NONE', *, *, #25827, .F. ) ;
#10002=AXIS2_PLACEMENT_3D ( 'NONE', #2880, #749, #12977 ) ;
#10006=ORIENTED_EDGE ( 'NONE', *, *, #2171, .F. ) ;
#10015=VECTOR ( 'NONE', #2873, 1000.000000000000000 ) ;
#10016=CIRCLE ( 'NONE', #13010, 69.99999999999998579 ) ;
#10034=ORIENTED_EDGE ( 'NONE', *, *, #25821, .F. ) ;
#10041=CARTESIAN_POINT ( 'NONE',  ( -210.0000000000000284, -66.50000000000001421, 66.50000000000005684 ) ) ;
#10044=VECTOR ( 'NONE', #8246, 1000.000000000000000 ) ;
#10066=AXIS2_PLACEMENT_3D ( 'NONE', #11472, #1001, #23222 ) ;
#10112=EDGE_CURVE ( 'NONE', #5117, #26151, #439, .T. ) ;
#10121=FACE_OUTER_BOUND ( 'NONE', #3045, .T. ) ;
#10128=VERTEX_POINT ( 'NONE', #6678 ) ;
#10132=CARTESIAN_POINT ( 'NONE',  ( -575.0231298121466352, 75.00000000000000000, -25.00000000000201794 ) ) ;
#10135=VERTEX_POINT ( 'NONE', #17058 ) ;
#10146=EDGE_CURVE ( 'NONE', #23489, #1760, #2962, .T. ) ;
#10148=AXIS2_PLACEMENT_3D ( 'NONE', #7572, #25444, #5721 ) ;
#10153=CARTESIAN_POINT ( 'NONE',  ( -639.5940242462432934, 29.29751003713100133, -27.23829469497263034 ) ) ;
#10154=CARTESIAN_POINT ( 'NONE',  ( -200.0000000000000284, 82.50000000000008527, 52.49999999999980105 ) ) ;
#10161=DIRECTION ( 'NONE',  ( 0.000000000000000000, 1.000000000000000000, 0.000000000000000000 ) ) ;
#10184=DIRECTION ( 'NONE',  ( 1.000000000000000000, 1.836970198721030427E-16, -0.000000000000000000 ) ) ;
#10191=AXIS2_PLACEMENT_3D ( 'NONE', #21611, #24239, #1890 ) ;
#10197=ORIENTED_EDGE ( 'NONE', *, *, #6969, .F. ) ;
#10201=APPLICATION_CONTEXT ( 'automotive_design' ) ;
#10207=EDGE_CURVE ( 'NONE', #19805, #4513, #13528, .T. ) ;
#10211=DIRECTION ( 'NONE',  ( 0.000000000000000000, 1.000000000000000000, 0.000000000000000000 ) ) ;
#10214=CARTESIAN_POINT ( 'NONE',  ( -678.9461782662789346, 75.00000000000000000, -24.99999999999826628 ) ) ;
#10245=CIRCLE ( 'NONE', #16183, 29.99999999999999645 ) ;
#10254=FACE_BOUND ( 'NONE', #13840, .T. ) ;
#10264=CARTESIAN_POINT ( 'NONE',  ( -266.9101291198153376, 0.000000000000000000, 0.000000000000000000 ) ) ;
#10271=VECTOR ( 'NONE', #7566, 1000.000000000000000 ) ;
#10277=LINE ( 'NONE', #24114, #9815 ) ;
#10294=CARTESIAN_POINT ( 'NONE',  ( -575.0231298121445889, 75.00000000000000000, 29.99999999999825206 ) ) ;
#10298=CARTESIAN_POINT ( 'NONE',  ( -678.9461782662789346, 90.00000000000000000, -34.99999999999845812 ) ) ;
#10307=VERTEX_POINT ( 'NONE', #18795 ) ;
#10314=CARTESIAN_POINT ( 'NONE',  ( -200.0000000000000000, 71.50000000000009948, 66.50000000000005684 ) ) ;
#10335=CARTESIAN_POINT ( 'NONE',  ( -626.9846540392142060, 75.00000000000000000, -60.00000000000000000 ) ) ;
#10406=DIRECTION ( 'NONE',  ( -1.000000000000000000, 0.000000000000000000, 0.000000000000000000 ) ) ;
#10410=CARTESIAN_POINT ( 'NONE',  ( -656.8721355146591350, 39.91566430679986865, -2.646366307133875218 ) ) ;
#10420=CARTESIAN_POINT ( 'NONE',  ( -631.7966154096428681, 28.60212811815375034, 34.74874185832601370 ) ) ;
#10433=CIRCLE ( 'NONE', #21889, 39.99999999999997158 ) ;
#10434=ADVANCED_FACE ( 'NONE', ( #19685 ), #10630, .F. ) ;
#10435=CIRCLE ( 'NONE', #9161, 39.99999999999991473 ) ;
#10515=DIRECTION ( 'NONE',  ( 0.000000000000000000, 0.000000000000000000, 1.000000000000000000 ) ) ;
#10536=ORIENTED_EDGE ( 'NONE', *, *, #21363, .F. ) ;
#10539=DIRECTION ( 'NONE',  ( -1.000000000000000000, 0.000000000000000000, 0.000000000000000000 ) ) ;
#10544=EDGE_CURVE ( 'NONE', #1596, #17045, #17408, .T. ) ;
#10547=CARTESIAN_POINT ( 'NONE',  ( -636.9543983739517898, 28.22693517060480772, 28.36072991200662941 ) ) ;
#10560=CARTESIAN_POINT ( 'NONE',  ( -594.0003854396136376, 43.45006682348635252, -11.76540767128717846 ) ) ;
#10567=DIRECTION ( 'NONE',  ( 0.000000000000000000, 1.000000000000000000, 0.000000000000000000 ) ) ;
#10595=EDGE_CURVE ( 'NONE', #19296, #13991, #9700, .T. ) ;
#10598=ADVANCED_FACE ( 'NONE', ( #5213 ), #15816, .T. ) ;
#10599=ORIENTED_EDGE ( 'NONE', *, *, #1126, .F. ) ;
#10612=CARTESIAN_POINT ( 'NONE',  ( -200.0000000000000000, -66.50000000000001421, 66.50000000000005684 ) ) ;
#10630=TOROIDAL_SURFACE ( 'NONE', #3345, 46.18033988749894547, 15.00000000000000000 ) ;
#10638=MECHANICAL_DESIGN_GEOMETRIC_PRESENTATION_REPRESENTATION('',(#18274),#8);
#10649=FACE_OUTER_BOUND ( 'NONE', #4914, .T. ) ;
#10680=AXIS2_PLACEMENT_3D ( 'NONE', #6129, #14111, #4014 ) ;
#10695=AXIS2_PLACEMENT_3D ( 'NONE', #23053, #8938, #14782 ) ;
#10697=CARTESIAN_POINT ( 'NONE',  ( -626.9846540392142060, 28.28427124746186649, 34.99999999999999289 ) ) ;
#10702=CARTESIAN_POINT ( 'NONE',  ( -597.5075361363678894, 40.84977275671060681, 18.90368210877456434 ) ) ;
#10707=ORIENTED_EDGE ( 'NONE', *, *, #3427, .T. ) ;
#10715=DIRECTION ( 'NONE',  ( -1.000000000000000000, 0.000000000000000000, 0.000000000000000000 ) ) ;
#10724=DIRECTION ( 'NONE',  ( -1.000000000000000000, -1.836970198721030181E-16, 0.000000000000000000 ) ) ;
#10734=ORIENTED_EDGE ( 'NONE', *, *, #6710, .F. ) ;
#10744=CARTESIAN_POINT ( 'NONE',  ( -626.9846540392097722, 75.00000000000000000, 65.00000000000002842 ) ) ;
#10760=VERTEX_POINT ( 'NONE', #8073 ) ;
#10790=CARTESIAN_POINT ( 'NONE',  ( -716.9846540392142060, 66.50000000000009948, 66.50000000000005684 ) ) ;
#10799=FACE_BOUND ( 'NONE', #19416, .T. ) ;
#10802=ORIENTED_EDGE ( 'NONE', *, *, #17433, .T. ) ;
#10814=CARTESIAN_POINT ( 'NONE',  ( -210.0000000000000284, 66.50000000000009948, 66.50000000000005684 ) ) ;
#10823=CARTESIAN_POINT ( 'NONE',  ( -626.9846540392142060, 95.00000000000000000, 0.000000000000000000 ) ) ;
#10827=CARTESIAN_POINT ( 'NONE',  ( -661.9859089885625281, 45.00097607149663048, -1.164717896653801654 ) ) ;
#10831=CARTESIAN_POINT ( 'NONE',  ( -596.9138871092466161, 41.28087457521051817, 17.94574729593260898 ) ) ;
#10836=ORIENTED_EDGE ( 'NONE', *, *, #2252, .F. ) ;
#10838=ORIENTED_EDGE ( 'NONE', *, *, #26318, .T. ) ;
#10842=DIRECTION ( 'NONE',  ( -1.000000000000000000, -1.836970198721030181E-16, 0.000000000000000000 ) ) ;
#10867=CYLINDRICAL_SURFACE ( 'NONE', #25560, 30.00000000000000000 ) ;
#10881=ADVANCED_FACE ( 'NONE', ( #21759 ), #7156, .F. ) ;
#10884=LINE ( 'NONE', #9134, #15917 ) ;
#10910=AXIS2_PLACEMENT_3D ( 'NONE', #22957, #5000, #11105 ) ;
#10927=ORIENTED_EDGE ( 'NONE', *, *, #14192, .T. ) ;
#10930=CARTESIAN_POINT ( 'NONE',  ( -716.9846540392142060, 66.50000000000009948, 66.50000000000005684 ) ) ;
#10941=ORIENTED_EDGE ( 'NONE', *, *, #4114, .F. ) ;
#10947=AXIS2_PLACEMENT_3D ( 'NONE', #6499, #12622, #526 ) ;
#10955=FACE_OUTER_BOUND ( 'NONE', #14523, .T. ) ;
#10968=CARTESIAN_POINT ( 'NONE',  ( -605.6399024805725730, 35.40302691160776050, 27.82394750457201127 ) ) ;
#10979=DIRECTION ( 'NONE',  ( 0.000000000000000000, 0.000000000000000000, 1.000000000000000000 ) ) ;
#10988=LINE ( 'NONE', #2609, #16382 ) ;
#10994=DIRECTION ( 'NONE',  ( 1.000000000000000000, 1.836970198721030427E-16, -0.000000000000000000 ) ) ;
#11000=CARTESIAN_POINT ( 'NONE',  ( -200.0000000000000000, 66.50000000000009948, 66.50000000000005684 ) ) ;
#11009=CIRCLE ( 'NONE', #822, 75.00000000000000000 ) ;
#11014=CARTESIAN_POINT ( 'NONE',  ( -716.9846540392142060, -52.49999999999991473, 82.49999999999998579 ) ) ;
#11023=EDGE_LOOP ( 'NONE', ( #24477, #5237, #2558, #10001 ) ) ;
#11042=CARTESIAN_POINT ( 'NONE',  ( -605.5768371412766555, 34.03271882474869159, 21.02205817263521226 ) ) ;
#11057=AXIS2_PLACEMENT_3D ( 'NONE', #17382, #25521, #23002 ) ;
#11061=ORIENTED_EDGE ( 'NONE', *, *, #6208, .T. ) ;
#11073=AXIS2_PLACEMENT_3D ( 'NONE', #16277, #8425, #6172 ) ;
#11089=CARTESIAN_POINT ( 'NONE',  ( -592.3042890440465271, 44.75177432878896155, -4.872409619293819105 ) ) ;
#11093=DIRECTION ( 'NONE',  ( 0.000000000000000000, -1.000000000000000000, 0.000000000000000000 ) ) ;
#11094=EDGE_LOOP ( 'NONE', ( #21206, #24113 ) ) ;
#11099=EDGE_CURVE ( 'NONE', #3746, #87, #20431, .T. ) ;
#11105=DIRECTION ( 'NONE',  ( 0.000000000000000000, 0.000000000000000000, 1.000000000000000000 ) ) ;
#11135=DIRECTION ( 'NONE',  ( 0.000000000000000000, 0.000000000000000000, 1.000000000000000000 ) ) ;
#11145=CARTESIAN_POINT ( 'NONE',  ( -200.0000000000000000, 52.49999999999987210, 82.49999999999998579 ) ) ;
#11163=CARTESIAN_POINT ( 'NONE',  ( -598.5566012994313496, 38.83482129691294205, 9.596881470589549323 ) ) ;
#11169=EDGE_CURVE ( 'NONE', #25214, #16256, #2077, .T. ) ;
#11180=VERTEX_POINT ( 'NONE', #18562 ) ;
#11181=ORIENTED_EDGE ( 'NONE', *, *, #6382, .F. ) ;
#11197=CARTESIAN_POINT ( 'NONE',  ( -716.9846540392142060, -82.49999999999991473, -52.49999999999977973 ) ) ;
#11211=DIRECTION ( 'NONE',  ( 0.000000000000000000, 1.000000000000000000, 0.000000000000000000 ) ) ;
#11212=CARTESIAN_POINT ( 'NONE',  ( -618.6895405067469937, 29.47063081262555784, 34.00782742777329304 ) ) ;
#11218=ORIENTED_EDGE ( 'NONE', *, *, #465, .F. ) ;
#11252=CARTESIAN_POINT ( 'NONE',  ( -652.7925989268254625, 36.95172673408348629, -15.41345145336517319 ) ) ;
#11277=PRODUCT_DEFINITION_FORMATION_WITH_SPECIFIED_SOURCE ( 'ANY', '', #3800, .NOT_KNOWN. ) ;
#11280=ADVANCED_FACE ( 'NONE', ( #4608 ), #25474, .T. ) ;
#11297=AXIS2_PLACEMENT_3D ( 'NONE', #16971, #4749, #2754 ) ;
#11304=EDGE_LOOP ( 'NONE', ( #24636, #13682 ) ) ;
#11331=CARTESIAN_POINT ( 'NONE',  ( -658.8956941877264626, 42.64142712027438620, -14.38834502120623249 ) ) ;
#11332=CARTESIAN_POINT ( 'NONE',  ( -726.9846540392142060, 52.49999999999991473, -82.49999999999998579 ) ) ;
#11335=DIRECTION ( 'NONE',  ( 0.000000000000000000, -1.000000000000000000, 0.000000000000000000 ) ) ;
#11336=AXIS2_PLACEMENT_3D ( 'NONE', #1184, #5295, #5052 ) ;
#11342=EDGE_LOOP ( 'NONE', ( #15263, #16946, #17103, #3330 ) ) ;
#11384=CARTESIAN_POINT ( 'NONE',  ( 0.000000000000000000, 0.000000000000000000, 0.000000000000000000 ) ) ;
#11388=EDGE_LOOP ( 'NONE', ( #22684, #7859, #23547, #9118 ) ) ;
#11393=EDGE_LOOP ( 'NONE', ( #17424, #6102, #10838, #20473 ) ) ;
#11397=VECTOR ( 'NONE', #3244, 1000.000000000000000 ) ;
#11401=DIRECTION ( 'NONE',  ( 0.000000000000000000, 1.000000000000000000, 0.000000000000000000 ) ) ;
#11404=EDGE_CURVE ( 'NONE', #16682, #17385, #1004, .T. ) ;
#11408=CARTESIAN_POINT ( 'NONE',  ( -599.5988719536647977, 38.07837741337411330, -12.25825338881973359 ) ) ;
#11418=VERTEX_POINT ( 'NONE', #17217 ) ;
#11424=EDGE_LOOP ( 'NONE', ( #16041, #9830 ) ) ;
#11427=DIRECTION ( 'NONE',  ( 0.000000000000000000, 1.000000000000000000, 0.000000000000000000 ) ) ;
#11428=AXIS2_PLACEMENT_3D ( 'NONE', #10790, #17028, #18900 ) ;
#11438=DIRECTION ( 'NONE',  ( 0.000000000000000000, 0.000000000000000000, 1.000000000000000000 ) ) ;
#11452=DIRECTION ( 'NONE',  ( 0.000000000000000000, 0.000000000000000000, 1.000000000000000000 ) ) ;
#11457=CARTESIAN_POINT ( 'NONE',  ( -625.7632191285248382, 28.30420643832251670, 34.98391645891658186 ) ) ;
#11472=CARTESIAN_POINT ( 'NONE',  ( -716.9846540392142060, -66.50000000000001421, -66.50000000000005684 ) ) ;
#11492=AXIS2_PLACEMENT_3D ( 'NONE', #9440, #1081, #25435 ) ;
#11497=CIRCLE ( 'NONE', #3444, 75.00000000000000000 ) ;
#11535=CARTESIAN_POINT ( 'NONE',  ( -626.9846540392142060, 26.45751311064579880, -30.00000000000005329 ) ) ;
#11548=ORIENTED_EDGE ( 'NONE', *, *, #19960, .T. ) ;
#11551=DIRECTION ( 'NONE',  ( 1.000000000000000000, 1.836970198721030427E-16, -0.000000000000000000 ) ) ;
#11552=LINE ( 'NONE', #15179, #8107 ) ;
#11553=ORIENTED_EDGE ( 'NONE', *, *, #13932, .T. ) ;
#11560=EDGE_CURVE ( 'NONE', #4752, #11180, #11009, .T. ) ;
#11582=ORIENTED_EDGE ( 'NONE', *, *, #23315, .F. ) ;
#11585=DIRECTION ( 'NONE',  ( 0.000000000000000000, 1.000000000000000000, 0.000000000000000000 ) ) ;
#11598=LINE ( 'NONE', #1639, #22754 ) ;
#11599=DIRECTION ( 'NONE',  ( -0.000000000000000000, -1.000000000000000000, -0.000000000000000000 ) ) ;
#11605=CARTESIAN_POINT ( 'NONE',  ( 0.000000000000000000, 0.000000000000000000, 0.000000000000000000 ) ) ;
#11620=EDGE_LOOP ( 'NONE', ( #24956, #21462, #14422, #10034 ) ) ;
#11623=CARTESIAN_POINT ( 'NONE',  ( -716.9846540392142060, 82.50000000000008527, 52.49999999999980105 ) ) ;
#11652=ORIENTED_EDGE ( 'NONE', *, *, #4789, .F. ) ;
#11687=ORIENTED_EDGE ( 'NONE', *, *, #9770, .T. ) ;
#11697=CIRCLE ( 'NONE', #6623, 5.000000000000004441 ) ;
#11708=CARTESIAN_POINT ( 'NONE',  ( -200.0000000000000000, -52.49999999999972999, -82.49999999999998579 ) ) ;
#11731=ORIENTED_EDGE ( 'NONE', *, *, #7828, .T. ) ;
#11740=DIRECTION ( 'NONE',  ( 0.000000000000000000, 1.000000000000000000, 0.000000000000000000 ) ) ;
#11743=CIRCLE ( 'NONE', #12611, 5.000000000000011546 ) ;
#11757=ADVANCED_FACE ( 'NONE', ( #20536 ), #5901, .F. ) ;
#11760=DIRECTION ( 'NONE',  ( 0.000000000000000000, 1.000000000000000000, 0.000000000000000000 ) ) ;
#11767=CIRCLE ( 'NONE', #10947, 29.99999999999999645 ) ;
#11805=CARTESIAN_POINT ( 'NONE',  ( -602.7677399305880499, 35.86505692559326519, -17.73308590989056555 ) ) ;
#11819=ORIENTED_EDGE ( 'NONE', *, *, #10146, .F. ) ;
#11822=VERTEX_POINT ( 'NONE', #24667 ) ;
#11825=AXIS2_PLACEMENT_3D ( 'NONE', #4435, #2432, #20399 ) ;
#11826=ORIENTED_EDGE ( 'NONE', *, *, #12006, .F. ) ;
#11851=EDGE_LOOP ( 'NONE', ( #13099, #5813 ) ) ;
#11852=CIRCLE ( 'NONE', #398, 5.000000000000039080 ) ;
#11856=DIRECTION ( 'NONE',  ( -1.000000000000000000, 0.000000000000000000, 0.000000000000000000 ) ) ;
#11870=AXIS2_PLACEMENT_3D ( 'NONE', #4780, #8888, #25134 ) ;
#11872=DIRECTION ( 'NONE',  ( 1.000000000000000000, 1.836970198721030427E-16, -0.000000000000000000 ) ) ;
#11893=CIRCLE ( 'NONE', #21255, 30.00000000000000355 ) ;
#11910=AXIS2_PLACEMENT_3D ( 'NONE', #23918, #16066, #1850 ) ;
#11952=DIRECTION ( 'NONE',  ( 0.000000000000000000, -1.000000000000000000, 0.000000000000000000 ) ) ;
#11955=ORIENTED_EDGE ( 'NONE', *, *, #21670, .T. ) ;
#11956=ORIENTED_EDGE ( 'NONE', *, *, #8591, .F. ) ;
#11959=ORIENTED_EDGE ( 'NONE', *, *, #16442, .T. ) ;
#11974=ADVANCED_FACE ( 'NONE', ( #6947 ), #17052, .F. ) ;
#11979=LINE ( 'NONE', #21964, #23243 ) ;
#11980=CARTESIAN_POINT ( 'NONE',  ( -716.9846540392142060, -52.49999999999991473, 82.49999999999998579 ) ) ;
#11987=CARTESIAN_POINT ( 'NONE',  ( -726.9846540392142060, 0.000000000000000000, -39.99999999999991473 ) ) ;
#11998=DIRECTION ( 'NONE',  ( -1.000000000000000000, 0.000000000000000000, 0.000000000000000000 ) ) ;
#12006=EDGE_CURVE ( 'NONE', #17304, #17170, #7661, .T. ) ;
#12012=CARTESIAN_POINT ( 'NONE',  ( -650.6015225192315938, 35.46186828486367659, -18.52428024556027353 ) ) ;
#12031=DIRECTION ( 'NONE',  ( -1.000000000000000000, 0.000000000000000000, 0.000000000000000000 ) ) ;
#12055=ORIENTED_EDGE ( 'NONE', *, *, #23092, .T. ) ;
#12086=DIRECTION ( 'NONE',  ( 0.000000000000000000, 0.000000000000000000, 1.000000000000000000 ) ) ;
#12089=EDGE_LOOP ( 'NONE', ( #16775, #8839, #14481, #11061, #23419, #25681, #7066, #22524 ) ) ;
#12092=EDGE_CURVE ( 'NONE', #23789, #23087, #978, .T. ) ;
#12112=FACE_BOUND ( 'NONE', #7272, .T. ) ;
#12123=DIRECTION ( 'NONE',  ( 0.000000000000000000, 0.000000000000000000, 1.000000000000000000 ) ) ;
#12130=AXIS2_PLACEMENT_3D ( 'NONE', #12539, #12679, #586 ) ;
#12132=LINE ( 'NONE', #17974, #20022 ) ;
#12134=ORIENTED_EDGE ( 'NONE', *, *, #21670, .F. ) ;
#12144=CARTESIAN_POINT ( 'NONE',  ( -632.0909954410809632, 26.92861902581830691, -29.57939079808245353 ) ) ;
#12156=AXIS2_PLACEMENT_3D ( 'NONE', #2102, #10211, #14329 ) ;
#12157=DIRECTION ( 'NONE',  ( 0.000000000000000000, 0.000000000000000000, 1.000000000000000000 ) ) ;
#12167=VECTOR ( 'NONE', #16128, 1000.000000000000000 ) ;
#12168=DIRECTION ( 'NONE',  ( -1.000000000000000000, 0.000000000000000000, 0.000000000000000000 ) ) ;
#12173=PLANE ( 'NONE',  #5348 ) ;
#12193=AXIS2_PLACEMENT_3D ( 'NONE', #2049, #24396, #40 ) ;
#12232=ADVANCED_FACE ( 'NONE', ( #24939 ), #15320, .T. ) ;
#12248=DIRECTION ( 'NONE',  ( -1.000000000000000000, 0.000000000000000000, 0.000000000000000000 ) ) ;
#12257=DIRECTION ( 'NONE',  ( 1.000000000000000000, -0.000000000000000000, -0.000000000000000000 ) ) ;
#12266=ORIENTED_EDGE ( 'NONE', *, *, #13619, .F. ) ;
#12276=CARTESIAN_POINT ( 'NONE',  ( -632.1051217044982877, 26.93102622738082630, 29.57723565074837069 ) ) ;
#12292=ORIENTED_EDGE ( 'NONE', *, *, #13997, .F. ) ;
#12293=EDGE_LOOP ( 'NONE', ( #15926, #7527, #23971, #11819 ) ) ;
#12298=DIRECTION ( 'NONE',  ( 0.000000000000000000, 0.000000000000000000, -1.000000000000000000 ) ) ;
#12299=DIRECTION ( 'NONE',  ( 0.000000000000000000, 0.000000000000000000, -1.000000000000000000 ) ) ;
#12308=DIRECTION ( 'NONE',  ( 1.000000000000000000, 1.836970198721030427E-16, -0.000000000000000000 ) ) ;
#12312=VECTOR ( 'NONE', #18232, 1000.000000000000000 ) ;
#12353=VERTEX_POINT ( 'NONE', #19830 ) ;
#12373=DIRECTION ( 'NONE',  ( -1.000000000000000000, 0.000000000000000000, 0.000000000000000000 ) ) ;
#12380=ORIENTED_EDGE ( 'NONE', *, *, #7828, .F. ) ;
#12385=LINE ( 'NONE', #10132, #24658 ) ;
#12386=FACE_OUTER_BOUND ( 'NONE', #9796, .T. ) ;
#12387=( LENGTH_UNIT ( ) NAMED_UNIT ( * ) SI_UNIT ( .MILLI., .METRE. ) );
#12389=ORIENTED_EDGE ( 'NONE', *, *, #22824, .T. ) ;
#12392=CARTESIAN_POINT ( 'NONE',  ( -716.9846540392142060, -66.50000000000001421, 71.50000000000005684 ) ) ;
#12414=CARTESIAN_POINT ( 'NONE',  ( -653.0498733801694016, 38.46191729815036808, 23.36466092414772078 ) ) ;
#12460=CARTESIAN_POINT ( 'NONE',  ( -575.0231298121466352, 90.00000000000000000, -35.00000000000203926 ) ) ;
#12476=ADVANCED_FACE ( 'NONE', ( #16503 ), #26245, .F. ) ;
#12482=ADVANCED_FACE ( 'NONE', ( #24366, #24499, #20370, #18493, #8248, #3739 ), #15964, .F. ) ;
#12483=ORIENTED_EDGE ( 'NONE', *, *, #3076, .T. ) ;
#12485=FACE_OUTER_BOUND ( 'NONE', #14952, .T. ) ;
#12486=ADVANCED_FACE ( 'NONE', ( #19965 ), #22239, .T. ) ;
#12502=DIRECTION ( 'NONE',  ( 1.000000000000000000, 1.836970198721030427E-16, -0.000000000000000000 ) ) ;
#12509=ORIENTED_EDGE ( 'NONE', *, *, #8329, .F. ) ;
#12511=CARTESIAN_POINT ( 'NONE',  ( -626.9846540392142060, 90.00000000000000000, 0.000000000000000000 ) ) ;
#12521=EDGE_LOOP ( 'NONE', ( #17543, #5577, #16782, #13977 ) ) ;
#12533=CARTESIAN_POINT ( 'NONE',  ( -211.2619052429883482, 0.000000000000000000, 0.000000000000000000 ) ) ;
#12539=CARTESIAN_POINT ( 'NONE',  ( -210.0000000000000568, 82.50000000000008527, 52.49999999999980105 ) ) ;
#12540=VECTOR ( 'NONE', #12031, 1000.000000000000000 ) ;
#12545=EDGE_CURVE ( 'NONE', #7420, #4513, #2019, .T. ) ;
#12548=CARTESIAN_POINT ( 'NONE',  ( -592.3028590817393706, 44.75291643641201489, 4.747045580819023947 ) ) ;
#12555=CIRCLE ( 'NONE', #5317, 30.00000000000005329 ) ;
#12556=AXIS2_PLACEMENT_3D ( 'NONE', #24418, #18686, #6443 ) ;
#12558=CARTESIAN_POINT ( 'NONE',  ( -726.9846540392142060, 66.50000000000009948, -71.50000000000005684 ) ) ;
#12562=CARTESIAN_POINT ( 'NONE',  ( -210.0000000000000284, -71.50000000000002842, -66.50000000000005684 ) ) ;
#12571=CIRCLE ( 'NONE', #9176, 29.99999999999999289 ) ;
#12575=ADVANCED_FACE ( 'NONE', ( #10121 ), #14502, .T. ) ;
#12576=EDGE_CURVE ( 'NONE', #1336, #16348, #3880, .T. ) ;
#12611=AXIS2_PLACEMENT_3D ( 'NONE', #14272, #2180, #3635 ) ;
#12622=DIRECTION ( 'NONE',  ( -1.000000000000000000, 0.000000000000000000, 0.000000000000000000 ) ) ;
#12649=VERTEX_POINT ( 'NONE', #22633 ) ;
#12651=DIRECTION ( 'NONE',  ( 0.000000000000000000, 0.000000000000000000, -1.000000000000000000 ) ) ;
#12658=DIRECTION ( 'NONE',  ( 1.000000000000000000, 1.836970198721030427E-16, -0.000000000000000000 ) ) ;
#12661=VERTEX_POINT ( 'NONE', #676 ) ;
#12668=CARTESIAN_POINT ( 'NONE',  ( -210.0000000000000284, 8.572527594031471415E-15, 69.99999999999998579 ) ) ;
#12672=CARTESIAN_POINT ( 'NONE',  ( -645.3052477932169495, 32.15456146116790848, 23.83018875450695617 ) ) ;
#12679=DIRECTION ( 'NONE',  ( 1.836970198721030427E-16, -1.000000000000000000, 0.000000000000000000 ) ) ;
#12681=CARTESIAN_POINT ( 'NONE',  ( -678.9461782662772293, 75.00000000000000000, 35.00000000000159162 ) ) ;
#12685=CARTESIAN_POINT ( 'NONE',  ( -593.9199682435015575, 43.50753815682832482, 11.70952539979739804 ) ) ;
#12686=ORIENTED_EDGE ( 'NONE', *, *, #17354, .F. ) ;
#12722=EDGE_CURVE ( 'NONE', #14871, #20514, #10245, .T. ) ;
#12728=EDGE_CURVE ( 'NONE', #2983, #18109, #19157, .T. ) ;
#12737=CIRCLE ( 'NONE', #5100, 5.000000000000095035 ) ;
#12759=CIRCLE ( 'NONE', #3008, 30.00000000000000000 ) ;
#12771=CARTESIAN_POINT ( 'NONE',  ( -598.7225062214002946, 38.71349023310503412, 10.07489800994831697 ) ) ;
#12782=ORIENTED_EDGE ( 'NONE', *, *, #23866, .T. ) ;
#12788=FACE_BOUND ( 'NONE', #15795, .T. ) ;
#12790=ORIENTED_EDGE ( 'NONE', *, *, #16780, .F. ) ;
#12791=ORIENTED_EDGE ( 'NONE', *, *, #19079, .T. ) ;
#12799=VECTOR ( 'NONE', #3455, 1000.000000000000000 ) ;
#12812=CARTESIAN_POINT ( 'NONE',  ( -648.4308094340339039, 34.05684324981173461, 20.98299627712672688 ) ) ;
#12819=FACE_OUTER_BOUND ( 'NONE', #5835, .T. ) ;
#12822=CARTESIAN_POINT ( 'NONE',  ( -660.1500850185274203, 43.58821494200376634, 11.19816822568961712 ) ) ;
#12826=CIRCLE ( 'NONE', #1343, 29.99999999999999289 ) ;
#12828=CARTESIAN_POINT ( 'NONE',  ( -617.0448027493109748, 29.97558630572889271, -33.56382543646817851 ) ) ;
#12833=ORIENTED_EDGE ( 'NONE', *, *, #21024, .F. ) ;
#12870=CARTESIAN_POINT ( 'NONE',  ( -575.0231298121445889, 75.00000000000000000, 29.99999999999825206 ) ) ;
#12905=DIRECTION ( 'NONE',  ( 1.000000000000000000, 0.000000000000000000, -0.000000000000000000 ) ) ;
#12927=EDGE_LOOP ( 'NONE', ( #15609, #26252, #25303, #20482 ) ) ;
#12931=ORIENTED_EDGE ( 'NONE', *, *, #19384, .T. ) ;
#12940=DIRECTION ( 'NONE',  ( 1.000000000000000000, 1.836970198721030427E-16, -0.000000000000000000 ) ) ;
#12941=CARTESIAN_POINT ( 'NONE',  ( -266.9101291198153376, 0.000000000000000000, 0.000000000000000000 ) ) ;
#12958=ORIENTED_EDGE ( 'NONE', *, *, #3151, .T. ) ;
#12977=DIRECTION ( 'NONE',  ( 0.000000000000000000, -1.000000000000000000, 0.000000000000000000 ) ) ;
#12985=CARTESIAN_POINT ( 'NONE',  ( -210.0000000000000284, -69.99999999999998579, 8.572527594031471415E-15 ) ) ;
#12993=CARTESIAN_POINT ( 'NONE',  ( -716.9846540392142060, 52.50000000000007816, 52.49999999999999289 ) ) ;
#13010=AXIS2_PLACEMENT_3D ( 'NONE', #3057, #13665, #19788 ) ;
#13021=AXIS2_PLACEMENT_3D ( 'NONE', #15918, #3699, #5827 ) ;
#13023=CARTESIAN_POINT ( 'NONE',  ( -678.9461782662789346, 75.00000000000000000, -34.99999999999845812 ) ) ;
#13026=ORIENTED_EDGE ( 'NONE', *, *, #24745, .F. ) ;
#13033=DIRECTION ( 'NONE',  ( 0.000000000000000000, 0.000000000000000000, 1.000000000000000000 ) ) ;
#13041=CARTESIAN_POINT ( 'NONE',  ( -620.4318289324395437, 27.25272540324414550, 29.27987691734877274 ) ) ;
#13059=EDGE_LOOP ( 'NONE', ( #14521, #18411 ) ) ;
#13084=CYLINDRICAL_SURFACE ( 'NONE', #25477, 75.00000000000000000 ) ;
#13091=CARTESIAN_POINT ( 'NONE',  ( -678.9461782662772293, 90.00000000000000000, 35.00000000000159162 ) ) ;
#13092=CARTESIAN_POINT ( 'NONE',  ( -591.9853919005129228, 44.99942610803522314, -0.6435327916369084633 ) ) ;
#13093=VERTEX_POINT ( 'NONE', #10154 ) ;
#13099=ORIENTED_EDGE ( 'NONE', *, *, #5110, .T. ) ;
#13108=DIRECTION ( 'NONE',  ( 1.000000000000000000, 1.836970198721030427E-16, -0.000000000000000000 ) ) ;
#13173=DIRECTION ( 'NONE',  ( -1.000000000000000000, 0.000000000000000000, 0.000000000000000000 ) ) ;
#13186=CARTESIAN_POINT ( 'NONE',  ( -716.9846540392142060, -82.49999999999991473, -52.49999999999977973 ) ) ;
#13188=ORIENTED_EDGE ( 'NONE', *, *, #25121, .F. ) ;
#13210=DIRECTION ( 'NONE',  ( 0.000000000000000000, 0.000000000000000000, -1.000000000000000000 ) ) ;
#13221=DIRECTION ( 'NONE',  ( 0.000000000000000000, 0.000000000000000000, 1.000000000000000000 ) ) ;
#13224=ORIENTED_EDGE ( 'NONE', *, *, #19519, .T. ) ;
#13228=DIRECTION ( 'NONE',  ( 0.000000000000000000, -1.000000000000000000, 0.000000000000000000 ) ) ;
#13245=ADVANCED_FACE ( 'NONE', ( #10955 ), #20026, .T. ) ;
#13249=AXIS2_PLACEMENT_3D ( 'NONE', #6899, #6635, #15016 ) ;
#13256=CARTESIAN_POINT ( 'NONE',  ( -628.0245654045285164, 26.47293912602897947, -29.98641569554063580 ) ) ;
#13263=VECTOR ( 'NONE', #2592, 1000.000000000000000 ) ;
#13298=DIRECTION ( 'NONE',  ( 1.000000000000000000, 1.836970198721030427E-16, -0.000000000000000000 ) ) ;
#13308=DIRECTION ( 'NONE',  ( 0.000000000000000000, -1.000000000000000000, 0.000000000000000000 ) ) ;
#13336=CARTESIAN_POINT ( 'NONE',  ( -575.0231298121466352, 75.00000000000000000, -30.00000000000202505 ) ) ;
#13360=DIRECTION ( 'NONE',  ( 0.000000000000000000, 1.000000000000000000, 0.000000000000000000 ) ) ;
#13365=ORIENTED_EDGE ( 'NONE', *, *, #21024, .T. ) ;
#13372=DIRECTION ( 'NONE',  ( 1.000000000000000000, -0.000000000000000000, -0.000000000000000000 ) ) ;
#13386=CARTESIAN_POINT ( 'NONE',  ( -716.9846540392142060, 82.50000000000008527, -52.49999999999977973 ) ) ;
#13393=ORIENTED_EDGE ( 'NONE', *, *, #3363, .F. ) ;
#13397=CARTESIAN_POINT ( 'NONE',  ( -210.0000000000000284, 52.50000000000007816, 52.49999999999999289 ) ) ;
#13398=EDGE_LOOP ( 'NONE', ( #18114, #16420, #15804, #18378 ) ) ;
#13407=DIRECTION ( 'NONE',  ( 0.000000000000000000, 1.000000000000000000, 0.000000000000000000 ) ) ;
#13436=VECTOR ( 'NONE', #16055, 1000.000000000000000 ) ;
#13438=CARTESIAN_POINT ( 'NONE',  ( -678.9461782662772293, 75.00000000000000000, 25.00000000000157385 ) ) ;
#13439=VECTOR ( 'NONE', #1880, 1000.000000000000000 ) ;
#13458=CARTESIAN_POINT ( 'NONE',  ( -655.1879134060876595, 39.94028867827254459, -20.75640583205202816 ) ) ;
#13467=DIRECTION ( 'NONE',  ( 0.000000000000000000, 0.000000000000000000, -1.000000000000000000 ) ) ;
#13468=ORIENTED_EDGE ( 'NONE', *, *, #18340, .F. ) ;
#13469=EDGE_LOOP ( 'NONE', ( #21940, #12509, #10802, #18954 ) ) ;
#13478=DIRECTION ( 'NONE',  ( 0.000000000000000000, -1.000000000000000000, 0.000000000000000000 ) ) ;
#13496=LINE ( 'NONE', #11623, #12540 ) ;
#13500=DIRECTION ( 'NONE',  ( 0.000000000000000000, 0.000000000000000000, 1.000000000000000000 ) ) ;
#13517=EDGE_LOOP ( 'NONE', ( #10836, #13393 ) ) ;
#13523=EDGE_CURVE ( 'NONE', #3113, #21007, #12826, .T. ) ;
#13528=CIRCLE ( 'NONE', #22906, 5.000000000000011546 ) ;
#13533=CARTESIAN_POINT ( 'NONE',  ( -626.9846540392142060, 90.00000000000000000, -46.18033988749894547 ) ) ;
#13537=CARTESIAN_POINT ( 'NONE',  ( -617.0486879783372842, 28.24773862521455214, -28.32390266690136471 ) ) ;
#13552=EDGE_LOOP ( 'NONE', ( #24201, #16551, #21707, #2733, #22080 ) ) ;
#13578=CARTESIAN_POINT ( 'NONE',  ( -661.3723022781085774, 44.52532212870602280, -6.545884190707156769 ) ) ;
#13582=DIRECTION ( 'NONE',  ( 0.000000000000000000, 0.000000000000000000, 1.000000000000000000 ) ) ;
#13583=FACE_OUTER_BOUND ( 'NONE', #11023, .T. ) ;
#13619=EDGE_CURVE ( 'NONE', #16348, #17701, #15561, .T. ) ;
#13624=AXIS2_PLACEMENT_3D ( 'NONE', #11384, #25645, #21390 ) ;
#13628=CIRCLE ( 'NONE', #4739, 5.000000000000039080 ) ;
#13629=DIRECTION ( 'NONE',  ( 0.000000000000000000, 1.000000000000000000, 0.000000000000000000 ) ) ;
#13640=LINE ( 'NONE', #13386, #8308 ) ;
#13651=CARTESIAN_POINT ( 'NONE',  ( -200.0000000000000000, -71.50000000000002842, 66.50000000000005684 ) ) ;
#13665=DIRECTION ( 'NONE',  ( 1.000000000000000000, -0.000000000000000000, -0.000000000000000000 ) ) ;
#13668=CARTESIAN_POINT ( 'NONE',  ( -611.0068738282783443, 30.90074614832916566, -25.40852347241385800 ) ) ;
#13682=ORIENTED_EDGE ( 'NONE', *, *, #21906, .T. ) ;
#13690=ORIENTED_EDGE ( 'NONE', *, *, #3427, .F. ) ;
#13706=LINE ( 'NONE', #3878, #10044 ) ;
#13749=FACE_OUTER_BOUND ( 'NONE', #15080, .T. ) ;
#13791=AXIS2_PLACEMENT_3D ( 'NONE', #22673, #20809, #4582 ) ;
#13793=CARTESIAN_POINT ( 'NONE',  ( -597.8200346137707584, 39.37724756625295441, -7.048631215857795951 ) ) ;
#13800=ORIENTED_EDGE ( 'NONE', *, *, #20172, .F. ) ;
#13815=AXIS2_PLACEMENT_3D ( 'NONE', #17651, #19656, #25411 ) ;
#13824=CIRCLE ( 'NONE', #246, 30.00000000000000000 ) ;
#13831=CARTESIAN_POINT ( 'NONE',  ( -626.9846540392142060, 75.00000000000000000, 0.000000000000000000 ) ) ;
#13840=EDGE_LOOP ( 'NONE', ( #24515, #1928 ) ) ;
#13843=CARTESIAN_POINT ( 'NONE',  ( -726.9846540392142060, 52.49999999999991473, -82.49999999999998579 ) ) ;
#13845=CARTESIAN_POINT ( 'NONE',  ( -716.9846540392142060, 66.50000000000009948, 71.50000000000005684 ) ) ;
#13850=CARTESIAN_POINT ( 'NONE',  ( -210.0000000000000284, 52.50000000000007816, -52.49999999999999289 ) ) ;
#13855=VERTEX_POINT ( 'NONE', #8741 ) ;
#13862=AXIS2_PLACEMENT_3D ( 'NONE', #10612, #102, #26204 ) ;
#13865=LINE ( 'NONE', #15722, #8310 ) ;
#13872=AXIS2_PLACEMENT_3D ( 'NONE', #21151, #19521, #13033 ) ;
#13906=DIRECTION ( 'NONE',  ( -1.000000000000000000, 0.000000000000000000, 0.000000000000000000 ) ) ;
#13913=ORIENTED_EDGE ( 'NONE', *, *, #21209, .T. ) ;
#13932=EDGE_CURVE ( 'NONE', #10135, #22711, #16719, .T. ) ;
#13961=DIRECTION ( 'NONE',  ( 0.000000000000000000, 0.000000000000000000, 1.000000000000000000 ) ) ;
#13964=FACE_BOUND ( 'NONE', #19672, .T. ) ;
#13968=FACE_BOUND ( 'NONE', #24411, .T. ) ;
#13970=DIRECTION ( 'NONE',  ( -0.000000000000000000, 0.000000000000000000, -1.000000000000000000 ) ) ;
#13977=ORIENTED_EDGE ( 'NONE', *, *, #11560, .T. ) ;
#13986=LINE ( 'NONE', #1496, #19807 ) ;
#13987=ORIENTED_EDGE ( 'NONE', *, *, #22836, .T. ) ;
#13989=CARTESIAN_POINT ( 'NONE',  ( -210.0000000000000284, -71.50000000000002842, 66.50000000000005684 ) ) ;
#13991=VERTEX_POINT ( 'NONE', #14987 ) ;
#13997=EDGE_CURVE ( 'NONE', #17170, #16549, #2857, .T. ) ;
#13998=FACE_BOUND ( 'NONE', #8094, .T. ) ;
#14002=CARTESIAN_POINT ( 'NONE',  ( -637.8274243086653996, 28.58169946791086957, -27.98848419961302980 ) ) ;
#14015=DIRECTION ( 'NONE',  ( 1.000000000000000000, 0.000000000000000000, -0.000000000000000000 ) ) ;
#14037=AXIS2_PLACEMENT_3D ( 'NONE', #14652, #25187, #7072 ) ;
#14039=CARTESIAN_POINT ( 'NONE',  ( -726.9846540392142060, -66.50000000000001421, 61.50000000000005684 ) ) ;
#14053=DIRECTION ( 'NONE',  ( 0.000000000000000000, 1.000000000000000000, 0.000000000000000000 ) ) ;
#14079=EDGE_LOOP ( 'NONE', ( #12292, #11826, #22343, #7688 ) ) ;
#14082=ORIENTED_EDGE ( 'NONE', *, *, #7691, .F. ) ;
#14109=DIRECTION ( 'NONE',  ( 0.000000000000000000, 0.000000000000000000, 1.000000000000000000 ) ) ;
#14111=DIRECTION ( 'NONE',  ( -0.000000000000000000, -1.000000000000000000, -0.000000000000000000 ) ) ;
#14115=CIRCLE ( 'NONE', #2664, 5.000000000000004441 ) ;
#14122=( NAMED_UNIT ( * ) SI_UNIT ( $, .STERADIAN. ) SOLID_ANGLE_UNIT ( ) );
#14129=ORIENTED_EDGE ( 'NONE', *, *, #10544, .T. ) ;
#14133=DIRECTION ( 'NONE',  ( 0.000000000000000000, 1.321694076934715579E-16, 1.000000000000000000 ) ) ;
#14135=FACE_OUTER_BOUND ( 'NONE', #20053, .T. ) ;
#14141=CARTESIAN_POINT ( 'NONE',  ( -678.9461782662789346, 75.00000000000000000, -29.99999999999836220 ) ) ;
#14146=CYLINDRICAL_SURFACE ( 'NONE', #25310, 69.99999999999998579 ) ;
#14147=DIRECTION ( 'NONE',  ( 1.836970198721030181E-16, -1.000000000000000000, 0.000000000000000000 ) ) ;
#14191=EDGE_CURVE ( 'NONE', #17701, #21989, #7481, .T. ) ;
#14192=EDGE_CURVE ( 'NONE', #5353, #20921, #1152, .T. ) ;
#14262=CARTESIAN_POINT ( 'NONE',  ( -716.9846540392142060, -66.50000000000001421, 61.50000000000005684 ) ) ;
#14263=AXIS2_PLACEMENT_3D ( 'NONE', #5099, #17319, #25452 ) ;
#14264=ADVANCED_FACE ( 'NONE', ( #19599, #17591 ), #17345, .F. ) ;
#14268=CARTESIAN_POINT ( 'NONE',  ( -629.0547673868355787, 26.53338973019900138, 29.93293935381844406 ) ) ;
#14272=CARTESIAN_POINT ( 'NONE',  ( -726.9846540392142060, 66.50000000000009948, -66.50000000000005684 ) ) ;
#14288=EDGE_LOOP ( 'NONE', ( #20954, #20210, #8840, #3754 ) ) ;
#14297=CYLINDRICAL_SURFACE ( 'NONE', #12556, 30.00000000000000000 ) ;
#14315=ORIENTED_EDGE ( 'NONE', *, *, #15160, .F. ) ;
#14320=VERTEX_POINT ( 'NONE', #25353 ) ;
#14321=DIRECTION ( 'NONE',  ( 0.000000000000000000, 1.000000000000000000, 0.000000000000000000 ) ) ;
#14322=VECTOR ( 'NONE', #253, 1000.000000000000000 ) ;
#14323=DIRECTION ( 'NONE',  ( 0.000000000000000000, 1.000000000000000000, 0.000000000000000000 ) ) ;
#14329=DIRECTION ( 'NONE',  ( 0.000000000000000000, 0.000000000000000000, 1.000000000000000000 ) ) ;
#14345=ADVANCED_FACE ( 'NONE', ( #15594 ), #25610, .F. ) ;
#14347=ORIENTED_EDGE ( 'NONE', *, *, #7424, .T. ) ;
#14350=ORIENTED_EDGE ( 'NONE', *, *, #16780, .T. ) ;
#14415=DIRECTION ( 'NONE',  ( -1.000000000000000000, 0.000000000000000000, 0.000000000000000000 ) ) ;
#14422=ORIENTED_EDGE ( 'NONE', *, *, #16234, .T. ) ;
#14430=CARTESIAN_POINT ( 'NONE',  ( -726.9846540392142060, 82.50000000000008527, 52.49999999999980105 ) ) ;
#14432=ADVANCED_FACE ( 'NONE', ( #7353 ), #15466, .T. ) ;
#14481=ORIENTED_EDGE ( 'NONE', *, *, #9480, .T. ) ;
#14493=AXIS2_PLACEMENT_3D ( 'NONE', #15703, #23827, #24100 ) ;
#14494=EDGE_CURVE ( 'NONE', #7095, #1180, #740, .T. ) ;
#14502=PLANE ( 'NONE',  #7251 ) ;
#14506=CARTESIAN_POINT ( 'NONE',  ( -716.9846540392142060, 82.50000000000008527, 52.49999999999980105 ) ) ;
#14516=ORIENTED_EDGE ( 'NONE', *, *, #2252, .T. ) ;
#14521=ORIENTED_EDGE ( 'NONE', *, *, #24689, .F. ) ;
#14523=EDGE_LOOP ( 'NONE', ( #7400, #19837, #1461, #20111 ) ) ;
#14530=EDGE_CURVE ( 'NONE', #4513, #19805, #11743, .T. ) ;
#14535=CARTESIAN_POINT ( 'NONE',  ( -627.5046577674308992, 26.45751311064576683, 30.00000000000004974 ) ) ;
#14545=CARTESIAN_POINT ( 'NONE',  ( -651.9208163904479534, 37.70578118159719594, 24.56594063796493543 ) ) ;
#14549=CARTESIAN_POINT ( 'NONE',  ( -617.6056806187223174, 29.79386004448080172, -33.72500239264033439 ) ) ;
#14609=ORIENTED_EDGE ( 'NONE', *, *, #19308, .T. ) ;
#14610=CARTESIAN_POINT ( 'NONE',  ( -716.9846540392142060, 66.50000000000009948, -71.50000000000005684 ) ) ;
#14612=EDGE_LOOP ( 'NONE', ( #8267, #15549 ) ) ;
#14632=FACE_OUTER_BOUND ( 'NONE', #11388, .T. ) ;
#14640=VERTEX_POINT ( 'NONE', #5098 ) ;
#14652=CARTESIAN_POINT ( 'NONE',  ( -210.0000000000000284, 0.000000000000000000, 0.000000000000000000 ) ) ;
#14676=CARTESIAN_POINT ( 'NONE',  ( -603.9947245077624984, 36.43016709300914613, -26.48061427247913002 ) ) ;
#14679=ADVANCED_FACE ( 'NONE', ( #20277, #2187, #23989, #8285, #26012, #18265 ), #17861, .T. ) ;
#14682=CARTESIAN_POINT ( 'NONE',  ( -210.0000000000000284, -52.49999999999991473, 82.49999999999998579 ) ) ;
#14688=CIRCLE ( 'NONE', #3224, 5.000000000000007994 ) ;
#14695=VECTOR ( 'NONE', #10406, 1000.000000000000000 ) ;
#14723=DIRECTION ( 'NONE',  ( 0.000000000000000000, 1.000000000000000000, 0.000000000000000000 ) ) ;
#14736=CIRCLE ( 'NONE', #2000, 5.000000000000046185 ) ;
#14749=CARTESIAN_POINT ( 'NONE',  ( -626.9846540392142060, 90.00000000000000000, 0.000000000000000000 ) ) ;
#14759=DIRECTION ( 'NONE',  ( 0.000000000000000000, 0.000000000000000000, 1.000000000000000000 ) ) ;
#14782=DIRECTION ( 'NONE',  ( 0.000000000000000000, 0.000000000000000000, -1.000000000000000000 ) ) ;
#14785=VERTEX_POINT ( 'NONE', #14506 ) ;
#14792=CARTESIAN_POINT ( 'NONE',  ( -210.0000000000000284, -61.50000000000001421, 66.50000000000005684 ) ) ;
#14796=CARTESIAN_POINT ( 'NONE',  ( -639.1748570899752622, 29.12792997464579869, 27.41590550727503839 ) ) ;
#14803=DIRECTION ( 'NONE',  ( 0.000000000000000000, 1.000000000000000000, 0.000000000000000000 ) ) ;
#14805=CARTESIAN_POINT ( 'NONE',  ( -639.6442031523718015, 30.97426854515512673, 32.64946120922897421 ) ) ;
#14809=CARTESIAN_POINT ( 'NONE',  ( -575.0231298121466352, 90.00000000000000000, -25.00000000000201794 ) ) ;
#14817=AXIS2_PLACEMENT_3D ( 'NONE', #12941, #24928, #710 ) ;
#14824=ADVANCED_FACE ( 'NONE', ( #6520, #25033, #6786, #4813, #6653, #2410 ), #680, .T. ) ;
#14871=VERTEX_POINT ( 'NONE', #4677 ) ;
#14877=CARTESIAN_POINT ( 'NONE',  ( -726.9846540392142060, -82.49999999999991473, -52.49999999999977973 ) ) ;
#14879=VECTOR ( 'NONE', #2030, 1000.000000000000000 ) ;
#14904=DIRECTION ( 'NONE',  ( -1.000000000000000000, 0.000000000000000000, 0.000000000000000000 ) ) ;
#14907=DIRECTION ( 'NONE',  ( 0.000000000000000000, 0.000000000000000000, 1.000000000000000000 ) ) ;
#14911=CARTESIAN_POINT ( 'NONE',  ( -210.0000000000000284, 71.50000000000011369, -66.50000000000005684 ) ) ;
#14923=CIRCLE ( 'NONE', #3442, 5.000000000000004441 ) ;
#14925=DIRECTION ( 'NONE',  ( 0.000000000000000000, 1.321694076934715579E-16, 1.000000000000000000 ) ) ;
#14936=DIRECTION ( 'NONE',  ( 0.000000000000000000, 1.000000000000000000, 0.000000000000000000 ) ) ;
#14941=CARTESIAN_POINT ( 'NONE',  ( -645.5937089524366002, 33.84884618228691977, 29.66287758167644384 ) ) ;
#14946=CARTESIAN_POINT ( 'NONE',  ( -600.8818656075578701, 38.48738506407975990, 23.32272707864667183 ) ) ;
#14952=EDGE_LOOP ( 'NONE', ( #18466, #15081, #4390, #13987 ) ) ;
#14987=CARTESIAN_POINT ( 'NONE',  ( -678.9461782662772293, 90.00000000000000000, 25.00000000000157385 ) ) ;
#15000=CARTESIAN_POINT ( 'NONE',  ( -575.0231298121445889, 75.00000000000000000, 34.99999999999821654 ) ) ;
#15009=DIRECTION ( 'NONE',  ( 1.000000000000000000, 1.836970198721030427E-16, -0.000000000000000000 ) ) ;
#15013=DIRECTION ( 'NONE',  ( 0.000000000000000000, -1.000000000000000000, 0.000000000000000000 ) ) ;
#15016=DIRECTION ( 'NONE',  ( 0.000000000000000000, -1.000000000000000000, 0.000000000000000000 ) ) ;
#15026=CARTESIAN_POINT ( 'NONE',  ( -608.6974641285738699, 32.13523715135190884, 23.85639593633560196 ) ) ;
#15048=ORIENTED_EDGE ( 'NONE', *, *, #4106, .T. ) ;
#15074=CARTESIAN_POINT ( 'NONE',  ( -607.9053911579920850, 34.11567477793045100, 29.34757030018079860 ) ) ;
#15080=EDGE_LOOP ( 'NONE', ( #12686, #6078, #11553, #24248 ) ) ;
#15081=ORIENTED_EDGE ( 'NONE', *, *, #5110, .F. ) ;
#15083=EDGE_CURVE ( 'NONE', #2915, #17336, #24632, .T. ) ;
#15120=CYLINDRICAL_SURFACE ( 'NONE', #16850, 4.999999999999962697 ) ;
#15126=AXIS2_PLACEMENT_3D ( 'NONE', #21072, #25205, #4981 ) ;
#15136=AXIS2_PLACEMENT_3D ( 'NONE', #21655, #9416, #5297 ) ;
#15142=DIRECTION ( 'NONE',  ( -1.000000000000000000, -1.836970198721030181E-16, 0.000000000000000000 ) ) ;
#15157=CARTESIAN_POINT ( 'NONE',  ( -602.8008298560588401, 35.84274269654262923, 17.77774983073336657 ) ) ;
#15160=EDGE_CURVE ( 'NONE', #17045, #1596, #14736, .T. ) ;
#15179=CARTESIAN_POINT ( 'NONE',  ( -210.0000000000000284, 52.49999999999987210, 82.49999999999998579 ) ) ;
#15181=VECTOR ( 'NONE', #20695, 1000.000000000000000 ) ;
#15202=CARTESIAN_POINT ( 'NONE',  ( -648.3187378681612927, 35.39633748653459122, -27.83271332065643122 ) ) ;
#15208=DIRECTION ( 'NONE',  ( -1.000000000000000000, 0.000000000000000000, 0.000000000000000000 ) ) ;
#15241=EDGE_CURVE ( 'NONE', #9502, #7420, #5394, .T. ) ;
#15244=CARTESIAN_POINT ( 'NONE',  ( -649.3705987078609496, 34.65645333158514774, -19.97733489359173120 ) ) ;
#15259=FACE_OUTER_BOUND ( 'NONE', #4987, .T. ) ;
#15263=ORIENTED_EDGE ( 'NONE', *, *, #1668, .F. ) ;
#15265=DIRECTION ( 'NONE',  ( -1.000000000000000000, 0.000000000000000000, 0.000000000000000000 ) ) ;
#15268=VERTEX_POINT ( 'NONE', #7550 ) ;
#15300=PLANE ( 'NONE',  #11492 ) ;
#15302=ORIENTED_EDGE ( 'NONE', *, *, #13619, .T. ) ;
#15320=CYLINDRICAL_SURFACE ( 'NONE', #918, 34.99999999999999289 ) ;
#15329=CYLINDRICAL_SURFACE ( 'NONE', #3500, 30.00000000000004974 ) ;
#15331=CARTESIAN_POINT ( 'NONE',  ( -609.3084111456423670, 33.35105114729260833, 30.21346475632024209 ) ) ;
#15367=VECTOR ( 'NONE', #10539, 1000.000000000000000 ) ;
#15374=CARTESIAN_POINT ( 'NONE',  ( -634.0640263162007386, 27.37139587162865340, -29.17014862255485852 ) ) ;
#15389=EDGE_LOOP ( 'NONE', ( #2065, #25432, #24, #7589 ) ) ;
#15420=EDGE_LOOP ( 'NONE', ( #18144, #24107, #16744, #2825 ) ) ;
#15421=ORIENTED_EDGE ( 'NONE', *, *, #19531, .T. ) ;
#15429=CARTESIAN_POINT ( 'NONE',  ( -716.9846540392142060, 52.49999999999991473, -82.49999999999998579 ) ) ;
#15442=CARTESIAN_POINT ( 'NONE',  ( -626.9846540392140923, 26.45751311064577749, 30.00000000000005329 ) ) ;
#15446=CARTESIAN_POINT ( 'NONE',  ( -649.9986597873944447, 36.44533412639378867, -26.46011044280707836 ) ) ;
#15448=CARTESIAN_POINT ( 'NONE',  ( -626.9846540392142060, 105.0000000000000000, 46.18033988749894547 ) ) ;
#15449=ORIENTED_EDGE ( 'NONE', *, *, #12722, .T. ) ;
#15454=DIRECTION ( 'NONE',  ( 0.000000000000000000, 0.000000000000000000, -1.000000000000000000 ) ) ;
#15457=VERTEX_POINT ( 'NONE', #3425 ) ;
#15462=EDGE_CURVE ( 'NONE', #7987, #3167, #17704, .T. ) ;
#15466=PLANE ( 'NONE',  #12193 ) ;
#15474=ADVANCED_FACE ( 'NONE', ( #19402 ), #17013, .T. ) ;
#15478=CARTESIAN_POINT ( 'NONE',  ( -678.9461782662772293, 75.00000000000000000, 30.00000000000158096 ) ) ;
#15501=DIRECTION ( 'NONE',  ( 0.000000000000000000, 0.000000000000000000, 1.000000000000000000 ) ) ;
#15502=CYLINDRICAL_SURFACE ( 'NONE', #25136, 5.000000000000011546 ) ;
#15508=ORIENTED_EDGE ( 'NONE', *, *, #2899, .T. ) ;
#15513=ORIENTED_EDGE ( 'NONE', *, *, #14530, .T. ) ;
#15524=CYLINDRICAL_SURFACE ( 'NONE', #1955, 30.00000000000000711 ) ;
#15527=CARTESIAN_POINT ( 'NONE',  ( -599.0136856033758477, 38.50067712691970456, -10.89074244889556731 ) ) ;
#15542=ORIENTED_EDGE ( 'NONE', *, *, #15241, .F. ) ;
#15546=LINE ( 'NONE', #7560, #12799 ) ;
#15549=ORIENTED_EDGE ( 'NONE', *, *, #21663, .T. ) ;
#15555=LINE ( 'NONE', #15429, #17436 ) ;
#15561=LINE ( 'NONE', #6339, #19600 ) ;
#15574=CARTESIAN_POINT ( 'NONE',  ( -661.6652239365027981, 44.75196652329666591, -4.756359218591798665 ) ) ;
#15576=ORIENTED_EDGE ( 'NONE', *, *, #24110, .T. ) ;
#15585=EDGE_LOOP ( 'NONE', ( #6759, #8090, #7466, #24813 ) ) ;
#15594=FACE_OUTER_BOUND ( 'NONE', #1753, .T. ) ;
#15605=CYLINDRICAL_SURFACE ( 'NONE', #25904, 5.000000000000095035 ) ;
#15609=ORIENTED_EDGE ( 'NONE', *, *, #6710, .T. ) ;
#15616=EDGE_CURVE ( 'NONE', #21778, #4752, #5022, .T. ) ;
#15653=DIRECTION ( 'NONE',  ( 0.000000000000000000, 0.000000000000000000, 1.000000000000000000 ) ) ;
#15654=CARTESIAN_POINT ( 'NONE',  ( -211.2619052429883482, 9.184850993605148733E-15, 75.00000000000000000 ) ) ;
#15656=CARTESIAN_POINT ( 'NONE',  ( -596.9857817216397962, 39.99915423894839250, 0.5766869916085746173 ) ) ;
#15672=LINE ( 'NONE', #23304, #8557 ) ;
#15685=DIRECTION ( 'NONE',  ( 0.000000000000000000, 1.000000000000000000, 0.000000000000000000 ) ) ;
#15699=CARTESIAN_POINT ( 'NONE',  ( -629.4336412755042147, 28.28427124746188071, -35.00000000000000000 ) ) ;
#15703=CARTESIAN_POINT ( 'NONE',  ( -575.0231298121445889, 90.00000000000000000, 29.99999999999825206 ) ) ;
#15704=CARTESIAN_POINT ( 'NONE',  ( -626.9846540392142060, 28.28427124746186649, 34.99999999999999289 ) ) ;
#15712=ORIENTED_EDGE ( 'NONE', *, *, #10207, .T. ) ;
#15722=CARTESIAN_POINT ( 'NONE',  ( -210.0000000000000284, -52.49999999999972999, -82.49999999999998579 ) ) ;
#15785=CARTESIAN_POINT ( 'NONE',  ( -597.0000841186025582, 39.98842450048364583, 1.092820868205398366 ) ) ;
#15793=EDGE_CURVE ( 'NONE', #2915, #10128, #19841, .T. ) ;
#15795=EDGE_LOOP ( 'NONE', ( #22217, #2247 ) ) ;
#15796=DIRECTION ( 'NONE',  ( 0.000000000000000000, -1.000000000000000000, 0.000000000000000000 ) ) ;
#15801=VERTEX_POINT ( 'NONE', #24007 ) ;
#15804=ORIENTED_EDGE ( 'NONE', *, *, #4263, .T. ) ;
#15816=PLANE ( 'NONE',  #24586 ) ;
#15830=VERTEX_POINT ( 'NONE', #3527 ) ;
#15834=DIRECTION ( 'NONE',  ( 0.000000000000000000, 1.000000000000000000, 0.000000000000000000 ) ) ;
#15836=( NAMED_UNIT ( * ) PLANE_ANGLE_UNIT ( ) SI_UNIT ( $, .RADIAN. ) );
#15840=DIRECTION ( 'NONE',  ( -1.000000000000000000, 0.000000000000000000, 0.000000000000000000 ) ) ;
#15848=CARTESIAN_POINT ( 'NONE',  ( -200.0000000000000284, 82.50000000000008527, 52.49999999999980105 ) ) ;
#15850=DIRECTION ( 'NONE',  ( 0.000000000000000000, 1.000000000000000000, 0.000000000000000000 ) ) ;
#15860=CARTESIAN_POINT ( 'NONE',  ( -210.0000000000000284, -52.49999999999992895, -52.49999999999999289 ) ) ;
#15882=EDGE_CURVE ( 'NONE', #4298, #25953, #19775, .T. ) ;
#15912=DIRECTION ( 'NONE',  ( 0.000000000000000000, 0.000000000000000000, -1.000000000000000000 ) ) ;
#15916=AXIS2_PLACEMENT_3D ( 'NONE', #24816, #12168, #2597 ) ;
#15917=VECTOR ( 'NONE', #18998, 1000.000000000000000 ) ;
#15918=CARTESIAN_POINT ( 'NONE',  ( -716.9846540392142060, -52.49999999999992895, -52.49999999999999289 ) ) ;
#15926=ORIENTED_EDGE ( 'NONE', *, *, #687, .F. ) ;
#15929=DIRECTION ( 'NONE',  ( 0.000000000000000000, 0.000000000000000000, -1.000000000000000000 ) ) ;
#15931=ORIENTED_EDGE ( 'NONE', *, *, #24689, .T. ) ;
#15935=VERTEX_POINT ( 'NONE', #5925 ) ;
#15951=ADVANCED_FACE ( 'NONE', ( #18151 ), #3398, .T. ) ;
#15953=CIRCLE ( 'NONE', #22790, 74.99999999999991473 ) ;
#15954=VECTOR ( 'NONE', #16275, 1000.000000000000000 ) ;
#15956=ORIENTED_EDGE ( 'NONE', *, *, #18880, .F. ) ;
#15964=PLANE ( 'NONE',  #19183 ) ;
#15977=DIRECTION ( 'NONE',  ( 1.000000000000000000, 0.000000000000000000, 0.000000000000000000 ) ) ;
#15981=FACE_OUTER_BOUND ( 'NONE', #9869, .T. ) ;
#15983=AXIS2_PLACEMENT_3D ( 'NONE', #10814, #12940, #2568 ) ;
#16008=CARTESIAN_POINT ( 'NONE',  ( -716.9846540392142060, -82.49999999999991473, -52.49999999999977973 ) ) ;
#16014=VERTEX_POINT ( 'NONE', #6183 ) ;
#16023=DIRECTION ( 'NONE',  ( 0.000000000000000000, 0.000000000000000000, 1.000000000000000000 ) ) ;
#16029=CARTESIAN_POINT ( 'NONE',  ( -626.9846540392142060, 90.00000000000000000, 74.99999999999991473 ) ) ;
#16031=CARTESIAN_POINT ( 'NONE',  ( -716.9846540392142060, -66.50000000000001421, -66.50000000000005684 ) ) ;
#16041=ORIENTED_EDGE ( 'NONE', *, *, #24118, .T. ) ;
#16047=ORIENTED_EDGE ( 'NONE', *, *, #19519, .F. ) ;
#16055=DIRECTION ( 'NONE',  ( 0.000000000000000000, 1.000000000000000000, 0.000000000000000000 ) ) ;
#16066=DIRECTION ( 'NONE',  ( -1.000000000000000000, -1.836970198721030181E-16, 0.000000000000000000 ) ) ;
#16073=VERTEX_POINT ( 'NONE', #4339 ) ;
#16097=CARTESIAN_POINT ( 'NONE',  ( -210.0000000000000284, 61.50000000000009237, -66.50000000000005684 ) ) ;
#16116=CYLINDRICAL_SURFACE ( 'NONE', #18753, 5.000000000000018652 ) ;
#16125=CIRCLE ( 'NONE', #16989, 74.99999999999991473 ) ;
#16128=DIRECTION ( 'NONE',  ( 0.000000000000000000, 1.000000000000000000, 0.000000000000000000 ) ) ;
#16145=EDGE_CURVE ( 'NONE', #21989, #9701, #604, .T. ) ;
#16147=EDGE_CURVE ( 'NONE', #6279, #15935, #314, .T. ) ;
#16179=CIRCLE ( 'NONE', #14493, 4.999999999999962697 ) ;
#16183=AXIS2_PLACEMENT_3D ( 'NONE', #2405, #8652, #10515 ) ;
#16185=TOROIDAL_SURFACE ( 'NONE', #18310, 46.18033988749894547, 15.00000000000000000 ) ;
#16214=ORIENTED_EDGE ( 'NONE', *, *, #24600, .F. ) ;
#16219=CIRCLE ( 'NONE', #23024, 46.18033988749894547 ) ;
#16220=CYLINDRICAL_SURFACE ( 'NONE', #24726, 5.000000000000004441 ) ;
#16231=DIRECTION ( 'NONE',  ( 0.000000000000000000, 1.000000000000000000, 0.000000000000000000 ) ) ;
#16234=EDGE_CURVE ( 'NONE', #21773, #9962, #11697, .T. ) ;
#16236=CARTESIAN_POINT ( 'NONE',  ( -678.9461782662789346, 75.00000000000000000, -34.99999999999845812 ) ) ;
#16244=EDGE_LOOP ( 'NONE', ( #15576, #8223 ) ) ;
#16248=( NAMED_UNIT ( * ) PLANE_ANGLE_UNIT ( ) SI_UNIT ( $, .RADIAN. ) );
#16256=VERTEX_POINT ( 'NONE', #10314 ) ;
#16259=CARTESIAN_POINT ( 'NONE',  ( -210.0000000000000000, -82.49999999999991473, -52.49999999999977973 ) ) ;
#16264=CARTESIAN_POINT ( 'NONE',  ( -652.2876273073196671, 36.60715735981532504, 16.14560165132014191 ) ) ;
#16275=DIRECTION ( 'NONE',  ( 0.000000000000000000, 1.000000000000000000, 0.000000000000000000 ) ) ;
#16277=CARTESIAN_POINT ( 'NONE',  ( -626.9846540392142060, 90.00000000000000000, 0.000000000000000000 ) ) ;
#16283=ORIENTED_EDGE ( 'NONE', *, *, #14191, .T. ) ;
#16284=EDGE_LOOP ( 'NONE', ( #8388, #4127 ) ) ;
#16303=CARTESIAN_POINT ( 'NONE',  ( -210.0000000000000284, 82.50000000000008527, -52.49999999999978684 ) ) ;
#16312=ORIENTED_EDGE ( 'NONE', *, *, #22658, .T. ) ;
#16318=EDGE_CURVE ( 'NONE', #19428, #14640, #22432, .T. ) ;
#16348=VERTEX_POINT ( 'NONE', #2205 ) ;
#16360=CARTESIAN_POINT ( 'NONE',  ( -626.9846540392142060, 75.00000000000000000, 0.000000000000000000 ) ) ;
#16364=DIRECTION ( 'NONE',  ( 0.000000000000000000, -0.000000000000000000, 1.000000000000000000 ) ) ;
#16375=DIRECTION ( 'NONE',  ( -1.000000000000000000, 0.000000000000000000, 0.000000000000000000 ) ) ;
#16382=VECTOR ( 'NONE', #19097, 1000.000000000000000 ) ;
#16410=CARTESIAN_POINT ( 'NONE',  ( -210.0000000000000284, 52.49999999999988631, -82.49999999999998579 ) ) ;
#16420=ORIENTED_EDGE ( 'NONE', *, *, #24303, .F. ) ;
#16421=EDGE_LOOP ( 'NONE', ( #12134, #5046 ) ) ;
#16422=ORIENTED_EDGE ( 'NONE', *, *, #1337, .T. ) ;
#16430=CARTESIAN_POINT ( 'NONE',  ( -726.9846540392142060, 66.50000000000009948, 66.50000000000005684 ) ) ;
#16438=CARTESIAN_POINT ( 'NONE',  ( -210.0000000000000284, -52.49999999999972999, -82.49999999999998579 ) ) ;
#16442=EDGE_CURVE ( 'NONE', #8666, #7950, #5361, .T. ) ;
#16456=AXIS2_PLACEMENT_3D ( 'NONE', #10335, #14321, #361 ) ;
#16482=EDGE_CURVE ( 'NONE', #8935, #4460, #15953, .T. ) ;
#16495=DIRECTION ( 'NONE',  ( 0.000000000000000000, 0.000000000000000000, 1.000000000000000000 ) ) ;
#16503=FACE_OUTER_BOUND ( 'NONE', #15420, .T. ) ;
#16512=CARTESIAN_POINT ( 'NONE',  ( -716.9846540392142060, 66.50000000000009948, 66.50000000000005684 ) ) ;
#16518=DIRECTION ( 'NONE',  ( 0.000000000000000000, 1.000000000000000000, 0.000000000000000000 ) ) ;
#16533=CARTESIAN_POINT ( 'NONE',  ( -640.9073278876498989, 29.89490142532471850, 26.57793756188680234 ) ) ;
#16549=VERTEX_POINT ( 'NONE', #13533 ) ;
#16551=ORIENTED_EDGE ( 'NONE', *, *, #465, .T. ) ;
#16568=DIRECTION ( 'NONE',  ( 0.000000000000000000, -1.000000000000000000, 0.000000000000000000 ) ) ;
#16581=ORIENTED_EDGE ( 'NONE', *, *, #4305, .T. ) ;
#16585=CIRCLE ( 'NONE', #14037, 69.99999999999998579 ) ;
#16624=AXIS2_PLACEMENT_3D ( 'NONE', #12533, #18659, #17062 ) ;
#16631=EDGE_CURVE ( 'NONE', #21007, #8002, #17056, .T. ) ;
#16641=VERTEX_POINT ( 'NONE', #18523 ) ;
#16645=DIRECTION ( 'NONE',  ( -1.000000000000000000, 0.000000000000000000, 0.000000000000000000 ) ) ;
#16647=ORIENTED_EDGE ( 'NONE', *, *, #17141, .T. ) ;
#16682=VERTEX_POINT ( 'NONE', #14792 ) ;
#16683=ORIENTED_EDGE ( 'NONE', *, *, #2899, .F. ) ;
#16699=CARTESIAN_POINT ( 'NONE',  ( -210.0000000000000284, 66.50000000000009948, 66.50000000000005684 ) ) ;
#16719=LINE ( 'NONE', #10744, #724 ) ;
#16736=VERTEX_POINT ( 'NONE', #12668 ) ;
#16744=ORIENTED_EDGE ( 'NONE', *, *, #4366, .T. ) ;
#16756=CARTESIAN_POINT ( 'NONE',  ( -726.9846540392142060, -52.49999999999991473, 52.49999999999999289 ) ) ;
#16765=CYLINDRICAL_SURFACE ( 'NONE', #22086, 4.999999999999997335 ) ;
#16770=DIRECTION ( 'NONE',  ( 0.000000000000000000, 1.000000000000000000, 0.000000000000000000 ) ) ;
#16775=ORIENTED_EDGE ( 'NONE', *, *, #13523, .T. ) ;
#16780=EDGE_CURVE ( 'NONE', #17459, #3571, #4834, .T. ) ;
#16782=ORIENTED_EDGE ( 'NONE', *, *, #15616, .T. ) ;
#16788=CYLINDRICAL_SURFACE ( 'NONE', #2594, 5.000000000000004441 ) ;
#16795=CARTESIAN_POINT ( 'NONE',  ( -648.7609290488377383, 34.26580538984126179, 20.64023319344268970 ) ) ;
#16802=DIRECTION ( 'NONE',  ( 1.000000000000000000, 1.836970198721030427E-16, -0.000000000000000000 ) ) ;
#16806=CARTESIAN_POINT ( 'NONE',  ( -659.5461728292011685, 43.13043488670722780, 12.84875797882843962 ) ) ;
#16810=CARTESIAN_POINT ( 'NONE',  ( -600.9160842859510012, 38.46169296933204862, -23.38072629326452301 ) ) ;
#16820=AXIS2_PLACEMENT_3D ( 'NONE', #19242, #23372, #25502 ) ;
#16829=VECTOR ( 'NONE', #14415, 1000.000000000000000 ) ;
#16850=AXIS2_PLACEMENT_3D ( 'NONE', #12870, #770, #4766 ) ;
#16851=ORIENTED_EDGE ( 'NONE', *, *, #16147, .F. ) ;
#16853=AXIS2_PLACEMENT_3D ( 'NONE', #10041, #24417, #9907 ) ;
#16879=ORIENTED_EDGE ( 'NONE', *, *, #5900, .F. ) ;
#16882=ADVANCED_FACE ( 'NONE', ( #25189 ), #6938, .F. ) ;
#16912=ORIENTED_EDGE ( 'NONE', *, *, #4305, .F. ) ;
#16916=ORIENTED_EDGE ( 'NONE', *, *, #4782, .T. ) ;
#16922=FACE_OUTER_BOUND ( 'NONE', #25599, .T. ) ;
#16925=DIRECTION ( 'NONE',  ( -1.000000000000000000, 0.000000000000000000, 0.000000000000000000 ) ) ;
#16929=CARTESIAN_POINT ( 'NONE',  ( -210.0000000000000284, -52.49999999999992895, -52.49999999999999289 ) ) ;
#16933=CARTESIAN_POINT ( 'NONE',  ( -210.0000000000000568, 82.50000000000008527, 52.49999999999980105 ) ) ;
#16941=CARTESIAN_POINT ( 'NONE',  ( -600.5150573586311111, 38.73722737577749342, 22.90562922617326080 ) ) ;
#16946=ORIENTED_EDGE ( 'NONE', *, *, #24784, .F. ) ;
#16971=CARTESIAN_POINT ( 'NONE',  ( -626.9846540392142060, 75.00000000000000000, -60.00000000000000000 ) ) ;
#16974=CIRCLE ( 'NONE', #8901, 34.99999999999999289 ) ;
#16979=DIRECTION ( 'NONE',  ( 0.000000000000000000, 0.000000000000000000, 1.000000000000000000 ) ) ;
#16989=AXIS2_PLACEMENT_3D ( 'NONE', #12511, #16770, #557 ) ;
#17013=CYLINDRICAL_SURFACE ( 'NONE', #11336, 75.00000000000000000 ) ;
#17022=CARTESIAN_POINT ( 'NONE',  ( -607.2519390358020246, 32.98910822842147894, 22.67520286530086793 ) ) ;
#17026=CARTESIAN_POINT ( 'NONE',  ( -210.0000000000000284, 69.99999999999998579, 0.000000000000000000 ) ) ;
#17028=DIRECTION ( 'NONE',  ( -1.000000000000000000, 0.000000000000000000, 0.000000000000000000 ) ) ;
#17033=VERTEX_POINT ( 'NONE', #19186 ) ;
#17042=ORIENTED_EDGE ( 'NONE', *, *, #21012, .T. ) ;
#17045=VERTEX_POINT ( 'NONE', #9073 ) ;
#17052=CONICAL_SURFACE ( 'NONE', #25546, 39.99999999999997158, 0.4944367829892074018 ) ;
#17056=LINE ( 'NONE', #18925, #1962 ) ;
#17058=CARTESIAN_POINT ( 'NONE',  ( -626.9846540392097722, 75.00000000000000000, 65.00000000000002842 ) ) ;
#17062=DIRECTION ( 'NONE',  ( 0.000000000000000000, 0.000000000000000000, -1.000000000000000000 ) ) ;
#17070=CARTESIAN_POINT ( 'NONE',  ( -652.3021900505264057, 37.95920247636578182, 24.17282378433309020 ) ) ;
#17071=CARTESIAN_POINT ( 'NONE',  ( -200.0000000000000000, 52.50000000000007816, 52.49999999999999289 ) ) ;
#17075=CARTESIAN_POINT ( 'NONE',  ( -593.2841520101219430, 43.99625175998158966, -9.521709705159564052 ) ) ;
#17076=ORIENTED_EDGE ( 'NONE', *, *, #545, .F. ) ;
#17103=ORIENTED_EDGE ( 'NONE', *, *, #25821, .T. ) ;
#17117=DIRECTION ( 'NONE',  ( 0.000000000000000000, 0.000000000000000000, -1.000000000000000000 ) ) ;
#17141=EDGE_CURVE ( 'NONE', #7950, #8666, #265, .T. ) ;
#17166=CARTESIAN_POINT ( 'NONE',  ( -266.9101291198153376, 5.510910596163085611E-15, 44.99999999999997158 ) ) ;
#17170=VERTEX_POINT ( 'NONE', #25661 ) ;
#17193=CARTESIAN_POINT ( 'NONE',  ( -660.7618416459580430, 44.05453155840947943, -9.478650601227100125 ) ) ;
#17198=DIRECTION ( 'NONE',  ( 0.000000000000000000, 0.000000000000000000, 1.000000000000000000 ) ) ;
#17208=ADVANCED_FACE ( 'NONE', ( #3428 ), #17648, .F. ) ;
#17217=CARTESIAN_POINT ( 'NONE',  ( -200.0000000000000000, -61.50000000000002132, -66.50000000000005684 ) ) ;
#17233=CARTESIAN_POINT ( 'NONE',  ( -716.9846540392142060, 0.000000000000000000, -44.99999999999997158 ) ) ;
#17238=CIRCLE ( 'NONE', #21081, 30.00000000000000355 ) ;
#17239=AXIS2_PLACEMENT_3D ( 'NONE', #23039, #18498, #4814 ) ;
#17246=ADVANCED_FACE ( 'NONE', ( #9675 ), #25536, .F. ) ;
#17250=CIRCLE ( 'NONE', #5780, 4.999999999999962697 ) ;
#17266=ORIENTED_EDGE ( 'NONE', *, *, #10146, .T. ) ;
#17276=DIRECTION ( 'NONE',  ( 0.000000000000000000, 1.000000000000000000, 0.000000000000000000 ) ) ;
#17282=CARTESIAN_POINT ( 'NONE',  ( -618.4965464916332394, 27.78215535369033873, 28.77840465361206412 ) ) ;
#17294=DIRECTION ( 'NONE',  ( 0.000000000000000000, 1.000000000000000000, 0.000000000000000000 ) ) ;
#17304=VERTEX_POINT ( 'NONE', #20325 ) ;
#17319=DIRECTION ( 'NONE',  ( -1.000000000000000000, 0.000000000000000000, 0.000000000000000000 ) ) ;
#17325=CARTESIAN_POINT ( 'NONE',  ( -660.0479240540959154, 43.50642481262257633, -11.71509576873842740 ) ) ;
#17326=DIRECTION ( 'NONE',  ( 0.000000000000000000, 1.000000000000000000, 0.000000000000000000 ) ) ;
#17336=VERTEX_POINT ( 'NONE', #12460 ) ;
#17337=UNCERTAINTY_MEASURE_WITH_UNIT (LENGTH_MEASURE( 1.000000000000000082E-05 ), #12387, 'distance_accuracy_value', 'NONE');
#17340=CARTESIAN_POINT ( 'NONE',  ( -716.9846540392142060, 5.510910596163085611E-15, 44.99999999999997158 ) ) ;
#17345=CYLINDRICAL_SURFACE ( 'NONE', #5809, 39.99999999999994316 ) ;
#17354=EDGE_CURVE ( 'NONE', #6105, #9566, #9939, .T. ) ;
#17362=LINE ( 'NONE', #25499, #4735 ) ;
#17369=CARTESIAN_POINT ( 'NONE',  ( -655.2474585732728656, 38.71397089290621807, -10.07298238254288769 ) ) ;
#17372=VECTOR ( 'NONE', #10184, 1000.000000000000000 ) ;
#17381=CYLINDRICAL_SURFACE ( 'NONE', #13624, 39.99999999999994316 ) ;
#17382=CARTESIAN_POINT ( 'NONE',  ( -210.0000000000000284, -66.50000000000001421, -66.50000000000005684 ) ) ;
#17385=VERTEX_POINT ( 'NONE', #5955 ) ;
#17394=AXIS2_PLACEMENT_3D ( 'NONE', #16512, #14904, #18638 ) ;
#17400=LINE ( 'NONE', #9419, #24912 ) ;
#17403=CARTESIAN_POINT ( 'NONE',  ( -601.6837166637907330, 36.60574833829470265, -16.14880282736276840 ) ) ;
#17408=CIRCLE ( 'NONE', #4634, 5.000000000000046185 ) ;
#17420=CARTESIAN_POINT ( 'NONE',  ( -678.9461782662789346, 75.00000000000000000, -29.99999999999836220 ) ) ;
#17424=ORIENTED_EDGE ( 'NONE', *, *, #3710, .F. ) ;
#17433=EDGE_CURVE ( 'NONE', #14785, #15268, #8072, .T. ) ;
#17434=EDGE_CURVE ( 'NONE', #2322, #12353, #19390, .T. ) ;
#17435=DIRECTION ( 'NONE',  ( 0.000000000000000000, 1.000000000000000000, 0.000000000000000000 ) ) ;
#17436=VECTOR ( 'NONE', #23680, 1000.000000000000000 ) ;
#17448=CARTESIAN_POINT ( 'NONE',  ( -654.5133026298142340, 39.46589736862178199, -21.64282600963380432 ) ) ;
#17459=VERTEX_POINT ( 'NONE', #5822 ) ;
#17460=CIRCLE ( 'NONE', #22146, 69.99999999999998579 ) ;
#17473=FACE_OUTER_BOUND ( 'NONE', #15389, .T. ) ;
#17500=AXIS2_PLACEMENT_3D ( 'NONE', #5487, #23339, #13221 ) ;
#17506=DIRECTION ( 'NONE',  ( 0.000000000000000000, 1.000000000000000000, 0.000000000000000000 ) ) ;
#17526=CYLINDRICAL_SURFACE ( 'NONE', #13815, 29.99999999999999645 ) ;
#17543=ORIENTED_EDGE ( 'NONE', *, *, #1337, .F. ) ;
#17545=DIRECTION ( 'NONE',  ( 0.000000000000000000, 0.000000000000000000, 1.000000000000000000 ) ) ;
#17556=CARTESIAN_POINT ( 'NONE',  ( -626.9846540392142060, 75.00000000000000000, 0.000000000000000000 ) ) ;
#17565=ADVANCED_FACE ( 'NONE', ( #4496 ), #15120, .F. ) ;
#17591=FACE_BOUND ( 'NONE', #22485, .T. ) ;
#17608=ORIENTED_EDGE ( 'NONE', *, *, #19953, .F. ) ;
#17634=ORIENTED_EDGE ( 'NONE', *, *, #23848, .T. ) ;
#17639=ORIENTED_EDGE ( 'NONE', *, *, #24784, .T. ) ;
#17648=CYLINDRICAL_SURFACE ( 'NONE', #4533, 5.000000000000046185 ) ;
#17651=CARTESIAN_POINT ( 'NONE',  ( -210.0000000000000284, -52.49999999999991473, 52.49999999999999289 ) ) ;
#17654=CARTESIAN_POINT ( 'NONE',  ( -600.4664386284592865, 37.45914613463217080, -14.03654238641473562 ) ) ;
#17662=ORIENTED_EDGE ( 'NONE', *, *, #8472, .T. ) ;
#17685=DIRECTION ( 'NONE',  ( 0.000000000000000000, -1.000000000000000000, 0.000000000000000000 ) ) ;
#17701=VERTEX_POINT ( 'NONE', #504 ) ;
#17704=CIRCLE ( 'NONE', #13872, 5.000000000000004441 ) ;
#17705=CYLINDRICAL_SURFACE ( 'NONE', #2144, 5.000000000000007994 ) ;
#17708=ORIENTED_EDGE ( 'NONE', *, *, #3969, .F. ) ;
#17734=DIRECTION ( 'NONE',  ( 0.000000000000000000, 0.000000000000000000, 1.000000000000000000 ) ) ;
#17794=VERTEX_POINT ( 'NONE', #3837 ) ;
#17807=ORIENTED_EDGE ( 'NONE', *, *, #8591, .T. ) ;
#17860=CARTESIAN_POINT ( 'NONE',  ( -716.9846540392142060, 66.50000000000009948, 61.50000000000005684 ) ) ;
#17861=PLANE ( 'NONE',  #6669 ) ;
#17871=DIRECTION ( 'NONE',  ( 0.000000000000000000, 0.000000000000000000, 1.000000000000000000 ) ) ;
#17875=CIRCLE ( 'NONE', #24268, 5.000000000000011546 ) ;
#17893=ADVANCED_FACE ( 'NONE', ( #25541 ), #3434, .T. ) ;
#17911=LINE ( 'NONE', #26054, #25531 ) ;
#17921=CARTESIAN_POINT ( 'NONE',  ( -613.0749189761168054, 29.88886548687010247, -26.58473085348082776 ) ) ;
#17938=ORIENTED_EDGE ( 'NONE', *, *, #6860, .T. ) ;
#17957=DIRECTION ( 'NONE',  ( -1.000000000000000000, 0.000000000000000000, 0.000000000000000000 ) ) ;
#17974=CARTESIAN_POINT ( 'NONE',  ( -265.6482238768269326, 0.000000000000000000, -39.99999999999997158 ) ) ;
#17991=PRODUCT_DEFINITION ( 'UNKNOWN', '', #11277, #19339 ) ;
#18034=ORIENTED_EDGE ( 'NONE', *, *, #21663, .F. ) ;
#18066=CARTESIAN_POINT ( 'NONE',  ( -210.0000000000000284, 0.000000000000000000, 0.000000000000000000 ) ) ;
#18069=ORIENTED_EDGE ( 'NONE', *, *, #20361, .T. ) ;
#18077=AXIS2_PLACEMENT_3D ( 'NONE', #21156, #4803, #12905 ) ;
#18081=ADVANCED_FACE ( 'NONE', ( #21298 ), #3073, .F. ) ;
#18108=CARTESIAN_POINT ( 'NONE',  ( -626.9846540392142060, 75.00000000000000000, -60.00000000000000000 ) ) ;
#18109=VERTEX_POINT ( 'NONE', #5573 ) ;
#18114=ORIENTED_EDGE ( 'NONE', *, *, #3781, .F. ) ;
#18122=FACE_OUTER_BOUND ( 'NONE', #23919, .T. ) ;
#18123=LINE ( 'NONE', #1910, #12167 ) ;
#18144=ORIENTED_EDGE ( 'NONE', *, *, #3151, .F. ) ;
#18151=FACE_OUTER_BOUND ( 'NONE', #21047, .T. ) ;
#18197=EDGE_LOOP ( 'NONE', ( #14609, #24917 ) ) ;
#18221=FACE_BOUND ( 'NONE', #21874, .T. ) ;
#18229=EDGE_LOOP ( 'NONE', ( #25236, #15542, #18772, #15712 ) ) ;
#18232=DIRECTION ( 'NONE',  ( 0.000000000000000000, -1.000000000000000000, 0.000000000000000000 ) ) ;
#18233=DIRECTION ( 'NONE',  ( 0.000000000000000000, -1.000000000000000000, 0.000000000000000000 ) ) ;
#18235=DIRECTION ( 'NONE',  ( 0.000000000000000000, 1.000000000000000000, 0.000000000000000000 ) ) ;
#18239=ORIENTED_EDGE ( 'NONE', *, *, #13997, .T. ) ;
#18241=DIRECTION ( 'NONE',  ( -1.000000000000000000, -1.836970198721030181E-16, 0.000000000000000000 ) ) ;
#18245=ORIENTED_EDGE ( 'NONE', *, *, #20785, .F. ) ;
#18264=CARTESIAN_POINT ( 'NONE',  ( -210.0000000000000284, -1.836970198721030378E-15, 0.000000000000000000 ) ) ;
#18265=FACE_BOUND ( 'NONE', #8431, .T. ) ;
#18267=DIRECTION ( 'NONE',  ( 0.000000000000000000, -0.000000000000000000, 1.000000000000000000 ) ) ;
#18274=STYLED_ITEM('',(#26374),#25811);
#18276=ORIENTED_EDGE ( 'NONE', *, *, #5393, .T. ) ;
#18303=CIRCLE ( 'NONE', #7671, 5.000000000000011546 ) ;
#18310=AXIS2_PLACEMENT_3D ( 'NONE', #22494, #404, #16495 ) ;
#18332=ORIENTED_EDGE ( 'NONE', *, *, #869, .F. ) ;
#18340=EDGE_CURVE ( 'NONE', #17033, #25214, #9019, .T. ) ;
#18368=AXIS2_PLACEMENT_3D ( 'NONE', #7464, #23702, #13582 ) ;
#18372=ORIENTED_EDGE ( 'NONE', *, *, #20350, .F. ) ;
#18378=ORIENTED_EDGE ( 'NONE', *, *, #12576, .T. ) ;
#18381=DIRECTION ( 'NONE',  ( 0.000000000000000000, -1.000000000000000000, 0.000000000000000000 ) ) ;
#18386=CARTESIAN_POINT ( 'NONE',  ( -199.9999999999999716, -82.49999999999991473, -52.49999999999977973 ) ) ;
#18393=CARTESIAN_POINT ( 'NONE',  ( -640.4792919554359969, 29.69771861375842192, 26.79787511901963271 ) ) ;
#18405=LINE ( 'NONE', #16008, #16829 ) ;
#18411=ORIENTED_EDGE ( 'NONE', *, *, #15882, .F. ) ;
#18419=FACE_OUTER_BOUND ( 'NONE', #21616, .T. ) ;
#18443=ORIENTED_EDGE ( 'NONE', *, *, #12092, .F. ) ;
#18466=ORIENTED_EDGE ( 'NONE', *, *, #15083, .F. ) ;
#18492=ADVANCED_FACE ( 'NONE', ( #20048 ), #20314, .F. ) ;
#18493=FACE_BOUND ( 'NONE', #4526, .T. ) ;
#18498=DIRECTION ( 'NONE',  ( 1.000000000000000000, 1.836970198721030427E-16, -0.000000000000000000 ) ) ;
#18510=CIRCLE ( 'NONE', #10002, 5.000000000000004441 ) ;
#18521=CIRCLE ( 'NONE', #2809, 74.99999999999991473 ) ;
#18523=CARTESIAN_POINT ( 'NONE',  ( -726.9846540392142060, -66.50000000000001421, -61.50000000000006395 ) ) ;
#18527=CARTESIAN_POINT ( 'NONE',  ( -646.7504686163034648, 33.00883640287656107, 22.64711897480060898 ) ) ;
#18528=CIRCLE ( 'NONE', #15126, 5.000000000000011546 ) ;
#18537=CARTESIAN_POINT ( 'NONE',  ( -657.0617608586776441, 41.27766484936599056, 18.03718546295864655 ) ) ;
#18545=CARTESIAN_POINT ( 'NONE',  ( -726.9846540392142060, -66.50000000000001421, -71.50000000000005684 ) ) ;
#18550=CIRCLE ( 'NONE', #8769, 5.000000000000039080 ) ;
#18562=CARTESIAN_POINT ( 'NONE',  ( -210.0000000000000284, 9.184850993605148733E-15, 75.00000000000000000 ) ) ;
#18580=VERTEX_POINT ( 'NONE', #18545 ) ;
#18604=ORIENTED_EDGE ( 'NONE', *, *, #1492, .F. ) ;
#18612=EDGE_LOOP ( 'NONE', ( #12380, #11959, #17807, #16214 ) ) ;
#18636=ORIENTED_EDGE ( 'NONE', *, *, #19706, .F. ) ;
#18638=DIRECTION ( 'NONE',  ( 0.000000000000000000, 0.000000000000000000, 1.000000000000000000 ) ) ;
#18647=EDGE_LOOP ( 'NONE', ( #1797, #16047, #419, #15931 ) ) ;
#18653=EDGE_CURVE ( 'NONE', #6362, #16256, #9858, .T. ) ;
#18658=CARTESIAN_POINT ( 'NONE',  ( -642.9707190394884719, 30.90505122157533435, 25.40327220459336388 ) ) ;
#18659=DIRECTION ( 'NONE',  ( 1.000000000000000000, -0.000000000000000000, -0.000000000000000000 ) ) ;
#18661=CIRCLE ( 'NONE', #22128, 5.000000000000007994 ) ;
#18666=DIRECTION ( 'NONE',  ( 1.000000000000000000, 1.836970198721030427E-16, -0.000000000000000000 ) ) ;
#18668=CARTESIAN_POINT ( 'NONE',  ( -635.2810310689012567, 29.45439800747776715, 34.02319262537031364 ) ) ;
#18673=CARTESIAN_POINT ( 'NONE',  ( -592.5938969088034582, 44.52772298657927763, 6.529736744792614900 ) ) ;
#18686=DIRECTION ( 'NONE',  ( -1.000000000000000000, 0.000000000000000000, 0.000000000000000000 ) ) ;
#18711=ORIENTED_EDGE ( 'NONE', *, *, #5910, .F. ) ;
#18731=EDGE_CURVE ( 'NONE', #12661, #5675, #20484, .T. ) ;
#18734=CARTESIAN_POINT ( 'NONE',  ( -626.9846540392142060, 75.00000000000000000, 0.000000000000000000 ) ) ;
#18736=EDGE_CURVE ( 'NONE', #21682, #5885, #6564, .T. ) ;
#18737=CARTESIAN_POINT ( 'NONE',  ( -210.0000000000000284, -61.50000000000002132, -66.50000000000005684 ) ) ;
#18738=ORIENTED_EDGE ( 'NONE', *, *, #6146, .T. ) ;
#18747=ORIENTED_EDGE ( 'NONE', *, *, #3782, .F. ) ;
#18753=AXIS2_PLACEMENT_3D ( 'NONE', #24246, #6019, #2699 ) ;
#18760=CARTESIAN_POINT ( 'NONE',  ( -597.8386401671281192, 39.36331430824176891, 7.179049609373510776 ) ) ;
#18771=ADVANCED_FACE ( 'NONE', ( #21214, #1375 ), #1116, .T. ) ;
#18772=ORIENTED_EDGE ( 'NONE', *, *, #21363, .T. ) ;
#18780=CIRCLE ( 'NONE', #19597, 5.000000000000004441 ) ;
#18790=LINE ( 'NONE', #22657, #15367 ) ;
#18795=CARTESIAN_POINT ( 'NONE',  ( -200.0000000000000000, 82.50000000000008527, -52.49999999999978684 ) ) ;
#18798=CARTESIAN_POINT ( 'NONE',  ( -628.0242092632672666, 26.47293101200708776, 29.98642280378765435 ) ) ;
#18812=CARTESIAN_POINT ( 'NONE',  ( -598.7739420286916356, 39.94555953491243372, 20.74621423265620379 ) ) ;
#18822=EDGE_CURVE ( 'NONE', #6493, #19428, #23868, .T. ) ;
#18849=CARTESIAN_POINT ( 'NONE',  ( -200.0000000000000000, -66.50000000000001421, -66.50000000000005684 ) ) ;
#18880=EDGE_CURVE ( 'NONE', #9962, #21773, #22195, .T. ) ;
#18900=DIRECTION ( 'NONE',  ( 0.000000000000000000, 0.000000000000000000, 1.000000000000000000 ) ) ;
#18910=PLANE ( 'NONE',  #692 ) ;
#18925=CARTESIAN_POINT ( 'NONE',  ( -210.0000000000000000, -82.49999999999991473, -52.49999999999977973 ) ) ;
#18940=VECTOR ( 'NONE', #18666, 1000.000000000000000 ) ;
#18942=CARTESIAN_POINT ( 'NONE',  ( -661.9254414355356175, 44.95389495940958824, -2.363913691310066234 ) ) ;
#18947=CARTESIAN_POINT ( 'NONE',  ( -605.6757189317567054, 35.38093617889416720, -27.85243504741141862 ) ) ;
#18953=ORIENTED_EDGE ( 'NONE', *, *, #2842, .T. ) ;
#18954=ORIENTED_EDGE ( 'NONE', *, *, #4120, .T. ) ;
#18960=DIRECTION ( 'NONE',  ( 0.000000000000000000, 1.000000000000000000, 0.000000000000000000 ) ) ;
#18966=DIRECTION ( 'NONE',  ( 0.000000000000000000, 1.000000000000000000, 0.000000000000000000 ) ) ;
#18976=CARTESIAN_POINT ( 'NONE',  ( -200.0000000000000000, -52.49999999999991473, 82.49999999999998579 ) ) ;
#18983=VERTEX_POINT ( 'NONE', #21909 ) ;
#18984=DIRECTION ( 'NONE',  ( 0.000000000000000000, 0.000000000000000000, 1.000000000000000000 ) ) ;
#18995=CARTESIAN_POINT ( 'NONE',  ( -575.0231298121466352, 75.00000000000000000, -30.00000000000202505 ) ) ;
#18998=DIRECTION ( 'NONE',  ( -0.000000000000000000, -1.000000000000000000, -0.000000000000000000 ) ) ;
#19028=CARTESIAN_POINT ( 'NONE',  ( -611.8588848697457934, 30.46712910405810959, 25.92524149612432893 ) ) ;
#19035=CARTESIAN_POINT ( 'NONE',  ( -726.9846540392142060, 39.99999999999991473, 0.000000000000000000 ) ) ;
#19045=ORIENTED_EDGE ( 'NONE', *, *, #18653, .F. ) ;
#19046=ORIENTED_EDGE ( 'NONE', *, *, #21498, .F. ) ;
#19047=CARTESIAN_POINT ( 'NONE',  ( -210.0000000000000284, -52.49999999999991473, 82.49999999999998579 ) ) ;
#19048=ORIENTED_EDGE ( 'NONE', *, *, #8097, .F. ) ;
#19076=CARTESIAN_POINT ( 'NONE',  ( -594.4172314860030610, 43.13402369259207347, -12.87267148120193383 ) ) ;
#19079=EDGE_CURVE ( 'NONE', #1336, #15830, #20178, .T. ) ;
#19097=DIRECTION ( 'NONE',  ( 0.000000000000000000, 1.000000000000000000, 0.000000000000000000 ) ) ;
#19103=CARTESIAN_POINT ( 'NONE',  ( -200.0000000000000000, -52.49999999999991473, 52.49999999999999289 ) ) ;
#19124=LINE ( 'NONE', #3030, #9204 ) ;
#19152=CARTESIAN_POINT ( 'NONE',  ( -614.3942928892040527, 29.28923948339344108, 27.24720710369317089 ) ) ;
#19157=LINE ( 'NONE', #17026, #24691 ) ;
#19180=AXIS2_PLACEMENT_3D ( 'NONE', #13850, #18241, #18381 ) ;
#19183=AXIS2_PLACEMENT_3D ( 'NONE', #9, #6003, #22105 ) ;
#19186=CARTESIAN_POINT ( 'NONE',  ( -210.0000000000000284, 61.50000000000009948, 66.50000000000005684 ) ) ;
#19198=CIRCLE ( 'NONE', #930, 4.999999999999997335 ) ;
#19200=CARTESIAN_POINT ( 'NONE',  ( -653.0828039730662340, 38.48173582175917318, -23.34791170400915306 ) ) ;
#19204=DIRECTION ( 'NONE',  ( -1.000000000000000000, 0.000000000000000000, 0.000000000000000000 ) ) ;
#19205=CARTESIAN_POINT ( 'NONE',  ( -595.2966944841457462, 42.47393186636156059, 14.90703951832045959 ) ) ;
#19211=ORIENTED_EDGE ( 'NONE', *, *, #5900, .T. ) ;
#19216=VECTOR ( 'NONE', #14053, 1000.000000000000000 ) ;
#19235=ORIENTED_EDGE ( 'NONE', *, *, #5121, .F. ) ;
#19242=CARTESIAN_POINT ( 'NONE',  ( -210.0000000000000284, 0.000000000000000000, 0.000000000000000000 ) ) ;
#19247=ADVANCED_FACE ( 'NONE', ( #23578 ), #21582, .T. ) ;
#19250=CARTESIAN_POINT ( 'NONE',  ( -266.9101291198153376, 0.000000000000000000, -44.99999999999997158 ) ) ;
#19296=VERTEX_POINT ( 'NONE', #13091 ) ;
#19307=CARTESIAN_POINT ( 'NONE',  ( -626.9846540392142060, 90.00000000000000000, -60.00000000000000000 ) ) ;
#19308=EDGE_CURVE ( 'NONE', #16073, #24029, #14115, .T. ) ;
#19326=CARTESIAN_POINT ( 'NONE',  ( -210.0000000000000284, -71.50000000000002842, -66.50000000000005684 ) ) ;
#19327=CARTESIAN_POINT ( 'NONE',  ( -623.9547998620685121, 28.43996653510315653, 34.87374174356184398 ) ) ;
#19339=PRODUCT_DEFINITION_CONTEXT ( 'detailed design', #21585, 'design' ) ;
#19348=CARTESIAN_POINT ( 'NONE',  ( -210.0000000000000284, -61.50000000000001421, 66.50000000000005684 ) ) ;
#19350=DIRECTION ( 'NONE',  ( 0.000000000000000000, 1.000000000000000000, 0.000000000000000000 ) ) ;
#19359=ORIENTED_EDGE ( 'NONE', *, *, #5571, .T. ) ;
#19361=CIRCLE ( 'NONE', #1103, 29.99999999999999289 ) ;
#19368=VECTOR ( 'NONE', #11551, 1000.000000000000000 ) ;
#19371=CARTESIAN_POINT ( 'NONE',  ( -653.7294268227522025, 37.61632567776710800, -13.73334781262508564 ) ) ;
#19384=EDGE_CURVE ( 'NONE', #15935, #6279, #958, .T. ) ;
#19390=CIRCLE ( 'NONE', #12156, 4.999999999999962697 ) ;
#19396=ADVANCED_FACE ( 'NONE', ( #1239 ), #15329, .F. ) ;
#19397=ORIENTED_EDGE ( 'NONE', *, *, #1492, .T. ) ;
#19400=CIRCLE ( 'NONE', #13862, 5.000000000000004441 ) ;
#19402=FACE_OUTER_BOUND ( 'NONE', #12521, .T. ) ;
#19416=EDGE_LOOP ( 'NONE', ( #20953, #23214 ) ) ;
#19423=ORIENTED_EDGE ( 'NONE', *, *, #14494, .F. ) ;
#19427=EDGE_LOOP ( 'NONE', ( #21672, #23143, #3415, #19045 ) ) ;
#19428=VERTEX_POINT ( 'NONE', #19326 ) ;
#19447=CARTESIAN_POINT ( 'NONE',  ( -635.2543834470891397, 29.44729488742095924, -34.02929410116306741 ) ) ;
#19494=DIRECTION ( 'NONE',  ( 0.000000000000000000, 0.000000000000000000, 1.000000000000000000 ) ) ;
#19504=AXIS2_PLACEMENT_3D ( 'NONE', #16699, #10724, #16568 ) ;
#19505=DIRECTION ( 'NONE',  ( 0.000000000000000000, 1.000000000000000000, 0.000000000000000000 ) ) ;
#19514=DIRECTION ( 'NONE',  ( 0.000000000000000000, 1.000000000000000000, 0.000000000000000000 ) ) ;
#19519=EDGE_CURVE ( 'NONE', #1180, #7095, #25195, .T. ) ;
#19521=DIRECTION ( 'NONE',  ( -1.000000000000000000, 0.000000000000000000, 0.000000000000000000 ) ) ;
#19524=DIRECTION ( 'NONE',  ( 0.000000000000000000, 0.000000000000000000, 1.000000000000000000 ) ) ;
#19530=CARTESIAN_POINT ( 'NONE',  ( -603.3435784881913833, 35.47800896442519303, -18.49335706250612077 ) ) ;
#19531=EDGE_CURVE ( 'NONE', #3571, #10760, #25847, .T. ) ;
#19548=DIRECTION ( 'NONE',  ( 0.000000000000000000, 1.000000000000000000, 0.000000000000000000 ) ) ;
#19551=ORIENTED_EDGE ( 'NONE', *, *, #2404, .F. ) ;
#19575=CARTESIAN_POINT ( 'NONE',  ( -658.6516411767275940, 42.45902836772346944, -14.91759928563551263 ) ) ;
#19580=DIRECTION ( 'NONE',  ( 0.000000000000000000, 0.000000000000000000, 1.000000000000000000 ) ) ;
#19582=CIRCLE ( 'NONE', #21712, 5.000000000000004441 ) ;
#19583=DIRECTION ( 'NONE',  ( 1.000000000000000000, -0.000000000000000000, -0.000000000000000000 ) ) ;
#19590=AXIS2_PLACEMENT_3D ( 'NONE', #17556, #21691, #13961 ) ;
#19597=AXIS2_PLACEMENT_3D ( 'NONE', #3725, #20089, #9971 ) ;
#19599=FACE_OUTER_BOUND ( 'NONE', #8134, .T. ) ;
#19600=VECTOR ( 'NONE', #9580, 1000.000000000000000 ) ;
#19656=DIRECTION ( 'NONE',  ( 1.000000000000000000, 1.836970198721030427E-16, -0.000000000000000000 ) ) ;
#19672=EDGE_LOOP ( 'NONE', ( #3581, #4332 ) ) ;
#19675=ORIENTED_EDGE ( 'NONE', *, *, #4120, .F. ) ;
#19685=FACE_OUTER_BOUND ( 'NONE', #20752, .T. ) ;
#19695=DIRECTION ( 'NONE',  ( -0.000000000000000000, -1.000000000000000000, -0.000000000000000000 ) ) ;
#19706=EDGE_CURVE ( 'NONE', #7498, #24112, #16179, .T. ) ;
#19707=CARTESIAN_POINT ( 'NONE',  ( -617.5592893540214163, 29.80849998618563745, 33.71207106400992615 ) ) ;
#19713=DIRECTION ( 'NONE',  ( 1.000000000000000000, -0.000000000000000000, -0.000000000000000000 ) ) ;
#19720=EDGE_CURVE ( 'NONE', #10307, #2553, #1761, .T. ) ;
#19728=CARTESIAN_POINT ( 'NONE',  ( -200.0000000000000000, -52.49999999999992895, -52.49999999999999289 ) ) ;
#19750=CARTESIAN_POINT ( 'NONE',  ( -678.9461782662789346, 90.00000000000000000, -29.99999999999836220 ) ) ;
#19770=EDGE_LOOP ( 'NONE', ( #6010, #19551, #1213, #12483 ) ) ;
#19775=CIRCLE ( 'NONE', #21912, 5.000000000000095035 ) ;
#19778=CIRCLE ( 'NONE', #4937, 5.000000000000007994 ) ;
#19784=CIRCLE ( 'NONE', #24482, 15.00000000000000000 ) ;
#19788=DIRECTION ( 'NONE',  ( 0.000000000000000000, 0.000000000000000000, -1.000000000000000000 ) ) ;
#19799=ORIENTED_EDGE ( 'NONE', *, *, #20058, .T. ) ;
#19805=VERTEX_POINT ( 'NONE', #22945 ) ;
#19807=VECTOR ( 'NONE', #6015, 1000.000000000000000 ) ;
#19830=CARTESIAN_POINT ( 'NONE',  ( -575.0231298121445889, 75.00000000000000000, 24.99999999999828759 ) ) ;
#19837=ORIENTED_EDGE ( 'NONE', *, *, #24600, .T. ) ;
#19841=CIRCLE ( 'NONE', #9170, 5.000000000000007994 ) ;
#19845=ORIENTED_EDGE ( 'NONE', *, *, #25121, .T. ) ;
#19855=EDGE_CURVE ( 'NONE', #567, #1760, #6017, .T. ) ;
#19866=DIRECTION ( 'NONE',  ( 0.000000000000000000, 0.000000000000000000, 1.000000000000000000 ) ) ;
#19887=EDGE_CURVE ( 'NONE', #7420, #9502, #18303, .T. ) ;
#19893=CARTESIAN_POINT ( 'NONE',  ( -265.6482238768269326, 0.000000000000000000, 0.000000000000000000 ) ) ;
#19908=VERTEX_POINT ( 'NONE', #13989 ) ;
#19920=CARTESIAN_POINT ( 'NONE',  ( -210.0000000000000284, 66.50000000000009948, -66.50000000000005684 ) ) ;
#19925=CARTESIAN_POINT ( 'NONE',  ( -596.9804635992022668, 40.00314282705044633, -1.996769250129288187 ) ) ;
#19953=EDGE_CURVE ( 'NONE', #16073, #7987, #160, .T. ) ;
#19955=VECTOR ( 'NONE', #11599, 1000.000000000000000 ) ;
#19960=EDGE_CURVE ( 'NONE', #87, #1721, #12132, .T. ) ;
#19962=FACE_BOUND ( 'NONE', #11304, .T. ) ;
#19964=EDGE_CURVE ( 'NONE', #23087, #1338, #22581, .T. ) ;
#19965=FACE_OUTER_BOUND ( 'NONE', #25469, .T. ) ;
#19987=LINE ( 'NONE', #14262, #23832 ) ;
#19990=CARTESIAN_POINT ( 'NONE',  ( -626.9846540392142060, 90.00000000000000000, 34.99999999999999289 ) ) ;
#20016=AXIS2_PLACEMENT_3D ( 'NONE', #11000, #893, #9003 ) ;
#20022=VECTOR ( 'NONE', #2163, 1000.000000000000000 ) ;
#20026=CONICAL_SURFACE ( 'NONE', #16624, 75.00000000000000000, 0.4944367829892072352 ) ;
#20037=LINE ( 'NONE', #24427, #5349 ) ;
#20045=VECTOR ( 'NONE', #1601, 1000.000000000000000 ) ;
#20048=FACE_OUTER_BOUND ( 'NONE', #3233, .T. ) ;
#20053=EDGE_LOOP ( 'NONE', ( #21216, #17938 ) ) ;
#20057=ADVANCED_FACE ( 'NONE', ( #15981 ), #16116, .F. ) ;
#20058=EDGE_CURVE ( 'NONE', #6112, #6279, #22912, .T. ) ;
#20075=ORIENTED_EDGE ( 'NONE', *, *, #20172, .T. ) ;
#20081=ORIENTED_EDGE ( 'NONE', *, *, #4263, .F. ) ;
#20089=DIRECTION ( 'NONE',  ( -1.000000000000000000, -1.836970198721030181E-16, 0.000000000000000000 ) ) ;
#20104=DIRECTION ( 'NONE',  ( -1.000000000000000000, 0.000000000000000000, 0.000000000000000000 ) ) ;
#20110=DIRECTION ( 'NONE',  ( 1.000000000000000000, -0.000000000000000000, -0.000000000000000000 ) ) ;
#20111=ORIENTED_EDGE ( 'NONE', *, *, #4779, .F. ) ;
#20127=DIRECTION ( 'NONE',  ( -1.000000000000000000, 0.000000000000000000, 0.000000000000000000 ) ) ;
#20132=CARTESIAN_POINT ( 'NONE',  ( -640.4516436576406022, 29.67861829237677540, -26.82428473879609143 ) ) ;
#20156=PRODUCT_DEFINITION_SHAPE ( 'NONE', 'NONE',  #17991 ) ;
#20172=EDGE_CURVE ( 'NONE', #21778, #2862, #23431, .T. ) ;
#20178=LINE ( 'NONE', #9931, #19216 ) ;
#20193=CIRCLE ( 'NONE', #13791, 4.999999999999962697 ) ;
#20210=ORIENTED_EDGE ( 'NONE', *, *, #8633, .F. ) ;
#20246=ORIENTED_EDGE ( 'NONE', *, *, #14530, .F. ) ;
#20248=CARTESIAN_POINT ( 'NONE',  ( -678.9461782662789346, 75.00000000000000000, -29.99999999999836220 ) ) ;
#20252=EDGE_LOOP ( 'NONE', ( #15048, #15421, #21584, #19359, #21428, #15302, #16283, #24550 ) ) ;
#20262=LINE ( 'NONE', #2041, #5559 ) ;
#20277=FACE_BOUND ( 'NONE', #3172, .T. ) ;
#20279=FACE_OUTER_BOUND ( 'NONE', #4957, .T. ) ;
#20296=UNCERTAINTY_MEASURE_WITH_UNIT (LENGTH_MEASURE( 1.000000000000000082E-05 ), #22388, 'distance_accuracy_value', 'NONE');
#20314=CYLINDRICAL_SURFACE ( 'NONE', #4795, 5.000000000000011546 ) ;
#20325=CARTESIAN_POINT ( 'NONE',  ( -626.9846540392142060, 95.00000000000000000, 34.99999999999999289 ) ) ;
#20350=EDGE_CURVE ( 'NONE', #23307, #26265, #17875, .T. ) ;
#20355=ADVANCED_FACE ( 'NONE', ( #21179 ), #15300, .F. ) ;
#20361=EDGE_CURVE ( 'NONE', #17033, #6362, #15546, .T. ) ;
#20370=FACE_BOUND ( 'NONE', #11094, .T. ) ;
#20398=EDGE_CURVE ( 'NONE', #17794, #24064, #11552, .T. ) ;
#20399=DIRECTION ( 'NONE',  ( 0.000000000000000000, -0.000000000000000000, 1.000000000000000000 ) ) ;
#20431=LINE ( 'NONE', #20702, #5890 ) ;
#20434=B_SPLINE_CURVE_WITH_KNOTS ( 'NONE', 3,
 ( #23080, #24809, #9092, #8966, #24675, #14549, #12828, #4588, #4852, #23205, #592, #20948, #8564, #18947, #14676, #8699, #16810, #22679, #24948, #4453, #21210, #2982, #2726, #19076, #10560, #17075, #20815, #857, #11089, #6696, #728, #22941, #13092, #20680, #25209, #6957, #12548, #2449, #18673, #22812, #12685, #19205, #2587, #10831, #10702, #18812, #8832, #16941, #14946, #4986, #21076, #2861, #10968, #15074, #987, #15331, #21710, #21337, #9470, #1240, #1494, #3108, #19707, #11212, #25336, #23579, #5483, #19327, #7592, #11457, #9600, #15704 ),
 .UNSPECIFIED., .F., .F.,
 ( 4, 2, 2, 2, 2, 2, 2, 2, 2, 2, 2, 2, 2, 2, 2, 2, 2, 2, 2, 2, 2, 2, 2, 2, 2, 2, 2, 2, 2, 2, 2, 2, 2, 2, 2, 4 ),
 ( 0.000000000000000000, 0.007188645765836454600, 0.008985807207295486501, 0.01078296864875452274, 0.01437729153167258654, 0.01797161441459064340, 0.02156593729750870547, 0.02875458306334482614, 0.03234890594626276678, 0.03414606738772174577, 0.03594322882918072476, 0.04313187459501699461, 0.04672619747793507056, 0.05032052036085313956, 0.05391484324377122245, 0.05571200468523027083, 0.05750916612668933309, 0.06110348900960745067, 0.06290065045106651986, 0.06469781189252560294, 0.07188645765836203239, 0.07548078054128025405, 0.07907510342419847571, 0.08266942630711668349, 0.08446658774857578045, 0.08626374919003489128, 0.09345239495587108480, 0.09524955639733019563, 0.09704671783878932034, 0.1006410407217078057, 0.1042353636046263049, 0.1060325250460855406, 0.1078296864875447902, 0.1114240093704632756, 0.1132211708119225391, 0.1150183322533817887 ),
 .UNSPECIFIED. ) ;
#20455=EDGE_CURVE ( 'NONE', #1338, #3113, #15672, .T. ) ;
#20473=ORIENTED_EDGE ( 'NONE', *, *, #11099, .F. ) ;
#20482=ORIENTED_EDGE ( 'NONE', *, *, #11404, .F. ) ;
#20484=CIRCLE ( 'NONE', #4772, 5.000000000000004441 ) ;
#20514=VERTEX_POINT ( 'NONE', #13186 ) ;
#20515=ORIENTED_EDGE ( 'NONE', *, *, #22985, .F. ) ;
#20520=ORIENTED_EDGE ( 'NONE', *, *, #6382, .T. ) ;
#20521=DIRECTION ( 'NONE',  ( 1.000000000000000000, 1.836970198721030427E-16, -0.000000000000000000 ) ) ;
#20536=FACE_OUTER_BOUND ( 'NONE', #8394, .T. ) ;
#20540=CARTESIAN_POINT ( 'NONE',  ( -659.3259227587273017, 42.96433640846947100, 13.39333494796945878 ) ) ;
#20548=ADVANCED_FACE ( 'NONE', ( #25528 ), #7277, .T. ) ;
#20552=ORIENTED_EDGE ( 'NONE', *, *, #5121, .T. ) ;
#20609=ORIENTED_EDGE ( 'NONE', *, *, #17433, .F. ) ;
#20625=PLANE ( 'NONE',  #1145 ) ;
#20637=ORIENTED_EDGE ( 'NONE', *, *, #25837, .T. ) ;
#20645=ORIENTED_EDGE ( 'NONE', *, *, #19953, .T. ) ;
#20646=CIRCLE ( 'NONE', #7459, 4.999999999999997335 ) ;
#20647=LINE ( 'NONE', #19047, #24926 ) ;
#20657=CARTESIAN_POINT ( 'NONE',  ( -626.9846540392142060, 75.00000000000000000, -74.99999999999991473 ) ) ;
#20660=AXIS2_PLACEMENT_3D ( 'NONE', #25989, #19583, #15454 ) ;
#20665=CARTESIAN_POINT ( 'NONE',  ( -656.9887313867761804, 40.00305800795492672, 2.000664094296076279 ) ) ;
#20673=DIRECTION ( 'NONE',  ( -1.000000000000000000, -1.836970198721030181E-16, 0.000000000000000000 ) ) ;
#20680=CARTESIAN_POINT ( 'NONE',  ( -591.9832520071217914, 45.00109046910024801, 1.162667027830338595 ) ) ;
#20688=CARTESIAN_POINT ( 'NONE',  ( -626.9846540392097722, 75.00000000000000000, 59.99999999999999289 ) ) ;
#20692=EDGE_CURVE ( 'NONE', #19908, #7220, #10277, .T. ) ;
#20695=DIRECTION ( 'NONE',  ( 1.000000000000000000, 1.836970198721030427E-16, -0.000000000000000000 ) ) ;
#20702=CARTESIAN_POINT ( 'NONE',  ( 0.000000000000000000, 0.000000000000000000, -39.99999999999994316 ) ) ;
#20716=AXIS2_PLACEMENT_3D ( 'NONE', #3801, #13629, #9909 ) ;
#20718=B_SPLINE_CURVE_WITH_KNOTS ( 'NONE', 3,
 ( #4806, #25414, #2806, #13041, #2676, #20763, #17282, #807, #6909, #19152, #4930, #19028, #8913, #15026, #17022, #11042, #937, #25285, #22889, #7041, #15157, #7165, #23284, #21286, #3060, #12771, #11163, #2533, #18760, #542, #24890, #6645, #20898, #15785, #15656, #19925, #9681, #23656, #13793, #25932, #3184, #1193, #15527, #11408, #9298, #5688, #17654, #3700, #17403, #11805, #19530, #1708, #7544, #21537, #25542, #13668, #1315, #17921, #25667, #5561, #3312, #5436, #13537, #21662, #9422, #3435, #23411, #11535 ),
 .UNSPECIFIED., .F., .F.,
 ( 4, 2, 2, 2, 2, 2, 2, 2, 2, 2, 2, 2, 2, 2, 2, 2, 2, 2, 2, 2, 2, 2, 2, 2, 2, 2, 2, 2, 2, 2, 2, 2, 2, 4 ),
 ( 1.132231036155057011E-16, 0.006124279316953675813, 0.007655349146192144856, 0.009186418975430613032, 0.01224855863390755806, 0.01531069829238450135, 0.01837283795086144464, 0.02449711726781507795, 0.02602818709705354006, 0.02755925692629199869, 0.03062139658476872861, 0.03674567590172217457, 0.03827674573096054300, 0.03980781556019890449, 0.04286995521867562747, 0.04593209487715235045, 0.04746316470639071194, 0.04899423453562907343, 0.05511851385258251246, 0.05664958368182088783, 0.05818065351105927707, 0.06124279316953602781, 0.06277386299877434073, 0.06430493282801265365, 0.06736707248648926560, 0.07042921214496587756, 0.07349135180344250340, 0.07961563112039596324, 0.08267777077887270010, 0.08420884060811119343, 0.08573991043734968676, 0.08880205009582670117, 0.09186418975430371558, 0.09798846907125773054 ),
 .UNSPECIFIED. ) ;
#20752=EDGE_LOOP ( 'NONE', ( #23585, #18239, #3238, #26214 ) ) ;
#20763=CARTESIAN_POINT ( 'NONE',  ( -618.9777491934191858, 27.63863534162878111, 28.91606862897691954 ) ) ;
#20785=EDGE_CURVE ( 'NONE', #24029, #16073, #19582, .T. ) ;
#20809=DIRECTION ( 'NONE',  ( 0.000000000000000000, 1.000000000000000000, 0.000000000000000000 ) ) ;
#20811=CARTESIAN_POINT ( 'NONE',  ( -638.5868188162663728, 30.55430815960217217, 33.04082901047623011 ) ) ;
#20815=CARTESIAN_POINT ( 'NONE',  ( -592.9819114055728733, 44.22852218735779672, -8.380006196786844441 ) ) ;
#20826=CARTESIAN_POINT ( 'NONE',  ( -626.9846540392142060, -82.50099999999990530, -30.00000000000004974 ) ) ;
#20851=VECTOR ( 'NONE', #21560, 1000.000000000000000 ) ;
#20867=ADVANCED_FACE ( 'NONE', ( #15259 ), #15502, .F. ) ;
#20870=ADVANCED_FACE ( 'NONE', ( #5162 ), #17381, .F. ) ;
#20876=AXIS2_PLACEMENT_3D ( 'NONE', #7953, #3987, #12086 ) ;
#20890=AXIS2_PLACEMENT_3D ( 'NONE', #4724, #2864, #4855 ) ;
#20898=CARTESIAN_POINT ( 'NONE',  ( -597.0557355404389455, 39.94671229542147017, 2.128033897213765790 ) ) ;
#20915=FACE_BOUND ( 'NONE', #18197, .T. ) ;
#20921=VERTEX_POINT ( 'NONE', #18386 ) ;
#20934=CARTESIAN_POINT ( 'NONE',  ( -631.0954681582677495, 26.75583256651325570, 29.73466928390865860 ) ) ;
#20940=DIRECTION ( 'NONE',  ( 0.000000000000000000, 0.000000000000000000, 1.000000000000000000 ) ) ;
#20944=CARTESIAN_POINT ( 'NONE',  ( -661.3556259495545646, 44.51244333536754993, 6.632513892488236529 ) ) ;
#20948=CARTESIAN_POINT ( 'NONE',  ( -609.3550727715755784, 33.31827460164921462, -30.25570868770995858 ) ) ;
#20953=ORIENTED_EDGE ( 'NONE', *, *, #15241, .T. ) ;
#20954=ORIENTED_EDGE ( 'NONE', *, *, #14191, .F. ) ;
#20980=FACE_OUTER_BOUND ( 'NONE', #14288, .T. ) ;
#20999=CARTESIAN_POINT ( 'NONE',  ( -716.9846540392142060, -66.50000000000001421, 61.50000000000005684 ) ) ;
#21004=CARTESIAN_POINT ( 'NONE',  ( -716.9846540392142060, -66.50000000000001421, -71.50000000000005684 ) ) ;
#21007=VERTEX_POINT ( 'NONE', #16259 ) ;
#21012=EDGE_CURVE ( 'NONE', #20921, #9153, #20262, .T. ) ;
#21024=EDGE_CURVE ( 'NONE', #24029, #3167, #19987, .T. ) ;
#21033=CARTESIAN_POINT ( 'NONE',  ( -210.0000000000000284, -66.50000000000001421, -66.50000000000005684 ) ) ;
#21047=EDGE_LOOP ( 'NONE', ( #16916, #1897, #19235, #24202 ) ) ;
#21056=CARTESIAN_POINT ( 'NONE',  ( -626.9846540392142060, -82.50099999999990530, 30.00000000000004974 ) ) ;
#21058=AXIS2_PLACEMENT_3D ( 'NONE', #7994, #22, #15977 ) ;
#21068=CIRCLE ( 'NONE', #15916, 4.999999999999997335 ) ;
#21071=DIRECTION ( 'NONE',  ( 0.000000000000000000, 0.000000000000000000, 1.000000000000000000 ) ) ;
#21072=CARTESIAN_POINT ( 'NONE',  ( -210.0000000000000284, 66.50000000000009948, -66.50000000000005684 ) ) ;
#21073=ORIENTED_EDGE ( 'NONE', *, *, #5562, .F. ) ;
#21076=CARTESIAN_POINT ( 'NONE',  ( -602.0130363958678572, 37.72923481230851195, 24.52994204380139109 ) ) ;
#21080=DIRECTION ( 'NONE',  ( -1.000000000000000000, -1.836970198721030181E-16, 0.000000000000000000 ) ) ;
#21081=AXIS2_PLACEMENT_3D ( 'NONE', #23886, #5663, #3673 ) ;
#21083=ORIENTED_EDGE ( 'NONE', *, *, #20058, .F. ) ;
#21137=DIRECTION ( 'NONE',  ( 0.000000000000000000, 0.000000000000000000, -1.000000000000000000 ) ) ;
#21151=CARTESIAN_POINT ( 'NONE',  ( -726.9846540392142060, -66.50000000000001421, 66.50000000000005684 ) ) ;
#21156=CARTESIAN_POINT ( 'NONE',  ( -210.0000000000000284, 52.49999999999988631, -82.49999999999998579 ) ) ;
#21176=ORIENTED_EDGE ( 'NONE', *, *, #13523, .F. ) ;
#21179=FACE_OUTER_BOUND ( 'NONE', #2950, .T. ) ;
#21185=EDGE_CURVE ( 'NONE', #14871, #10760, #18790, .T. ) ;
#21204=CARTESIAN_POINT ( 'NONE',  ( -636.3947065546303747, 29.79081638863893744, -33.73087704270072607 ) ) ;
#21206=ORIENTED_EDGE ( 'NONE', *, *, #8097, .T. ) ;
#21208=DIRECTION ( 'NONE',  ( 0.000000000000000000, 0.000000000000000000, 1.000000000000000000 ) ) ;
#21209=EDGE_CURVE ( 'NONE', #23307, #13991, #702, .T. ) ;
#21210=CARTESIAN_POINT ( 'NONE',  ( -598.4915613741692368, 40.14731501344079589, -20.33361824257625372 ) ) ;
#21214=FACE_BOUND ( 'NONE', #21935, .T. ) ;
#21216=ORIENTED_EDGE ( 'NONE', *, *, #12006, .T. ) ;
#21217=ORIENTED_EDGE ( 'NONE', *, *, #26177, .F. ) ;
#21255=AXIS2_PLACEMENT_3D ( 'NONE', #1757, #11856, #23964 ) ;
#21271=EDGE_LOOP ( 'NONE', ( #1079, #22785, #1401, #2858, #13690, #19046, #18711, #6204 ) ) ;
#21286=CARTESIAN_POINT ( 'NONE',  ( -599.2626224583869998, 38.32091463456419689, 11.47750068289685821 ) ) ;
#21289=VECTOR ( 'NONE', #12248, 1000.000000000000000 ) ;
#21298=FACE_OUTER_BOUND ( 'NONE', #12927, .T. ) ;
#21319=CARTESIAN_POINT ( 'NONE',  ( -726.9846540392142060, 66.50000000000009948, -66.50000000000005684 ) ) ;
#21336=CARTESIAN_POINT ( 'NONE',  ( -200.0000000000000000, 66.50000000000009948, -66.50000000000005684 ) ) ;
#21337=CARTESIAN_POINT ( 'NONE',  ( -611.2495423974685309, 32.35569666353303120, 31.28312433736698495 ) ) ;
#21347=LINE ( 'NONE', #3117, #7437 ) ;
#21348=AXIS2_PLACEMENT_3D ( 'NONE', #4458, #21080, #2453 ) ;
#21363=EDGE_CURVE ( 'NONE', #9502, #19805, #21814, .T. ) ;
#21379=CARTESIAN_POINT ( 'NONE',  ( -642.1214326342156937, 30.47265398018172888, -25.91871900570560783 ) ) ;
#21390=DIRECTION ( 'NONE',  ( 0.000000000000000000, 0.000000000000000000, -1.000000000000000000 ) ) ;
#21399=VERTEX_POINT ( 'NONE', #5586 ) ;
#21428=ORIENTED_EDGE ( 'NONE', *, *, #3781, .T. ) ;
#21432=EDGE_CURVE ( 'NONE', #26151, #2862, #23432, .T. ) ;
#21452=CARTESIAN_POINT ( 'NONE',  ( -652.3345777734953117, 37.97727100629618491, -24.15733517944065412 ) ) ;
#21459=CARTESIAN_POINT ( 'NONE',  ( -210.0000000000000284, 71.50000000000011369, -66.50000000000005684 ) ) ;
#21462=ORIENTED_EDGE ( 'NONE', *, *, #1668, .T. ) ;
#21463=ORIENTED_EDGE ( 'NONE', *, *, #5754, .T. ) ;
#21466=CARTESIAN_POINT ( 'NONE',  ( -726.9846540392142060, 82.50000000000008527, -52.49999999999977973 ) ) ;
#21470=AXIS2_PLACEMENT_3D ( 'NONE', #24538, #20673, #6294 ) ;
#21477=CYLINDRICAL_SURFACE ( 'NONE', #4922, 5.000000000000039080 ) ;
#21498=EDGE_CURVE ( 'NONE', #5885, #24064, #25439, .T. ) ;
#21500=CIRCLE ( 'NONE', #24923, 30.00000000000000355 ) ;
#21504=CARTESIAN_POINT ( 'NONE',  ( -646.7283122382513056, 32.99571033938487830, -22.66550611626425038 ) ) ;
#21514=DIRECTION ( 'NONE',  ( -1.000000000000000000, 0.000000000000000000, 0.000000000000000000 ) ) ;
#21537=CARTESIAN_POINT ( 'NONE',  ( -607.2237257255731038, 33.00592889815013109, -22.65123783916381939 ) ) ;
#21552=EDGE_LOOP ( 'NONE', ( #24341, #13468 ) ) ;
#21555=EDGE_LOOP ( 'NONE', ( #5981, #7816, #5546, #4859 ) ) ;
#21560=DIRECTION ( 'NONE',  ( 0.000000000000000000, 1.000000000000000000, 0.000000000000000000 ) ) ;
#21567=DIRECTION ( 'NONE',  ( 0.000000000000000000, 1.000000000000000000, 0.000000000000000000 ) ) ;
#21582=CYLINDRICAL_SURFACE ( 'NONE', #4354, 74.99999999999991473 ) ;
#21584=ORIENTED_EDGE ( 'NONE', *, *, #7357, .T. ) ;
#21585=APPLICATION_CONTEXT ( 'automotive_design' ) ;
#21611=CARTESIAN_POINT ( 'NONE',  ( 0.000000000000000000, 0.000000000000000000, 0.000000000000000000 ) ) ;
#21616=EDGE_LOOP ( 'NONE', ( #23364, #3996, #25265, #8866 ) ) ;
#21636=ADVANCED_FACE ( 'NONE', ( #9839 ), #16220, .F. ) ;
#21637=CARTESIAN_POINT ( 'NONE',  ( -716.9846540392142060, 66.50000000000009948, -66.50000000000005684 ) ) ;
#21655=CARTESIAN_POINT ( 'NONE',  ( -716.9846540392142060, 0.000000000000000000, 0.000000000000000000 ) ) ;
#21662=CARTESIAN_POINT ( 'NONE',  ( -618.9247522084408502, 27.64368523546104939, -28.91374874216926116 ) ) ;
#21663=EDGE_CURVE ( 'NONE', #7220, #17385, #18780, .T. ) ;
#21670=EDGE_CURVE ( 'NONE', #16641, #18580, #19198, .T. ) ;
#21672=ORIENTED_EDGE ( 'NONE', *, *, #20361, .F. ) ;
#21676=CIRCLE ( 'NONE', #8949, 5.000000000000004441 ) ;
#21682=VERTEX_POINT ( 'NONE', #21949 ) ;
#21691=DIRECTION ( 'NONE',  ( 0.000000000000000000, 1.000000000000000000, 0.000000000000000000 ) ) ;
#21705=CARTESIAN_POINT ( 'NONE',  ( -657.8774556453281548, 41.88472458230610584, -16.46082976225948613 ) ) ;
#21707=ORIENTED_EDGE ( 'NONE', *, *, #9011, .T. ) ;
#21710=CARTESIAN_POINT ( 'NONE',  ( -609.7891919193333479, 33.09846309977769607, 30.48971931906038435 ) ) ;
#21712=AXIS2_PLACEMENT_3D ( 'NONE', #7644, #7522, #21897 ) ;
#21745=EDGE_LOOP ( 'NONE', ( #19845, #1692 ) ) ;
#21759=FACE_OUTER_BOUND ( 'NONE', #13552, .T. ) ;
#21766=DIRECTION ( 'NONE',  ( 0.8802361161597901384, 0.000000000000000000, -0.4745359626076072757 ) ) ;
#21773=VERTEX_POINT ( 'NONE', #1868 ) ;
#21778=VERTEX_POINT ( 'NONE', #22487 ) ;
#21788=DIRECTION ( 'NONE',  ( 1.000000000000000000, 1.836970198721030427E-16, -0.000000000000000000 ) ) ;
#21814=LINE ( 'NONE', #1087, #20045 ) ;
#21846=CARTESIAN_POINT ( 'NONE',  ( -626.9846540392097722, 75.00000000000000000, 54.99999999999995737 ) ) ;
#21874=EDGE_LOOP ( 'NONE', ( #11652, #17076 ) ) ;
#21876=CYLINDRICAL_SURFACE ( 'NONE', #5679, 5.000000000000039080 ) ;
#21889=AXIS2_PLACEMENT_3D ( 'NONE', #7333, #5351, #13210 ) ;
#21897=DIRECTION ( 'NONE',  ( 0.000000000000000000, 0.000000000000000000, 1.000000000000000000 ) ) ;
#21906=EDGE_CURVE ( 'NONE', #16549, #7651, #16219, .T. ) ;
#21909=CARTESIAN_POINT ( 'NONE',  ( -626.9846540392142060, 28.28427124746186649, 34.99999999999999289 ) ) ;
#21912=AXIS2_PLACEMENT_3D ( 'NONE', #19750, #26163, #16023 ) ;
#21922=AXIS2_PLACEMENT_3D ( 'NONE', #17071, #9215, #7211 ) ;
#21935=EDGE_LOOP ( 'NONE', ( #7687, #8030 ) ) ;
#21940=ORIENTED_EDGE ( 'NONE', *, *, #16145, .F. ) ;
#21949=CARTESIAN_POINT ( 'NONE',  ( -210.0000000000000284, -52.49999999999991473, 82.49999999999998579 ) ) ;
#21964=CARTESIAN_POINT ( 'NONE',  ( -726.9846540392142060, -82.49999999999991473, -52.49999999999977973 ) ) ;
#21989=VERTEX_POINT ( 'NONE', #8770 ) ;
#21990=ORIENTED_EDGE ( 'NONE', *, *, #532, .F. ) ;
#22040=LINE ( 'NONE', #5534, #6186 ) ;
#22042=AXIS2_PLACEMENT_3D ( 'NONE', #19893, #1678, #24153 ) ;
#22049=DIRECTION ( 'NONE',  ( 0.000000000000000000, 1.000000000000000000, 0.000000000000000000 ) ) ;
#22061=CARTESIAN_POINT ( 'NONE',  ( -626.9846540392097722, 75.00000000000000000, 54.99999999999995737 ) ) ;
#22077=EDGE_CURVE ( 'NONE', #11822, #18109, #9001, .T. ) ;
#22080=ORIENTED_EDGE ( 'NONE', *, *, #19960, .F. ) ;
#22086=AXIS2_PLACEMENT_3D ( 'NONE', #21033, #6521, #24505 ) ;
#22099=FACE_BOUND ( 'NONE', #11851, .T. ) ;
#22103=PLANE ( 'NONE',  #9220 ) ;
#22105=DIRECTION ( 'NONE',  ( 1.836970198721030181E-16, -1.000000000000000000, 0.000000000000000000 ) ) ;
#22113=CYLINDRICAL_SURFACE ( 'NONE', #10191, 44.99999999999997158 ) ;
#22118=DIRECTION ( 'NONE',  ( 0.000000000000000000, 0.000000000000000000, 1.000000000000000000 ) ) ;
#22128=AXIS2_PLACEMENT_3D ( 'NONE', #22850, #14323, #16979 ) ;
#22129=PLANE ( 'NONE',  #11825 ) ;
#22132=CARTESIAN_POINT ( 'NONE',  ( -645.2837021124099692, 32.14196927292066874, -23.84742176288152748 ) ) ;
#22146=AXIS2_PLACEMENT_3D ( 'NONE', #18066, #7813, #15929 ) ;
#22151=ORIENTED_EDGE ( 'NONE', *, *, #4782, .F. ) ;
#22153=CIRCLE ( 'NONE', #20016, 5.000000000000004441 ) ;
#22163=DIRECTION ( 'NONE',  ( 0.000000000000000000, 1.000000000000000000, 0.000000000000000000 ) ) ;
#22184=ORIENTED_EDGE ( 'NONE', *, *, #10112, .F. ) ;
#22185=CARTESIAN_POINT ( 'NONE',  ( -678.9461782662772293, 75.00000000000000000, 30.00000000000158096 ) ) ;
#22189=ORIENTED_EDGE ( 'NONE', *, *, #21185, .T. ) ;
#22195=CIRCLE ( 'NONE', #17500, 5.000000000000004441 ) ;
#22217=ORIENTED_EDGE ( 'NONE', *, *, #17141, .F. ) ;
#22220=ORIENTED_EDGE ( 'NONE', *, *, #23866, .F. ) ;
#22222=DIRECTION ( 'NONE',  ( 0.000000000000000000, 1.000000000000000000, 0.000000000000000000 ) ) ;
#22233=EDGE_CURVE ( 'NONE', #6105, #10135, #11852, .T. ) ;
#22239=CYLINDRICAL_SURFACE ( 'NONE', #10680, 34.99999999999999289 ) ;
#22248=LINE ( 'NONE', #22386, #2971 ) ;
#22252=DIRECTION ( 'NONE',  ( 0.000000000000000000, 1.000000000000000000, 0.000000000000000000 ) ) ;
#22259=ORIENTED_EDGE ( 'NONE', *, *, #26072, .F. ) ;
#22263=ADVANCED_FACE ( 'NONE', ( #1274 ), #25630, .F. ) ;
#22281=LINE ( 'NONE', #1921, #15954 ) ;
#22288=ORIENTED_EDGE ( 'NONE', *, *, #10112, .T. ) ;
#22343=ORIENTED_EDGE ( 'NONE', *, *, #3626, .T. ) ;
#22356=ORIENTED_EDGE ( 'NONE', *, *, #6146, .F. ) ;
#22359=VECTOR ( 'NONE', #17326, 1000.000000000000000 ) ;
#22372=DIRECTION ( 'NONE',  ( 0.000000000000000000, -0.000000000000000000, 1.000000000000000000 ) ) ;
#22386=CARTESIAN_POINT ( 'NONE',  ( 0.000000000000000000, 4.898587196589405926E-15, 39.99999999999994316 ) ) ;
#22388=( LENGTH_UNIT ( ) NAMED_UNIT ( * ) SI_UNIT ( .MILLI., .METRE. ) );
#22391=ORIENTED_EDGE ( 'NONE', *, *, #24303, .T. ) ;
#22396=AXIS2_PLACEMENT_3D ( 'NONE', #4894, #9012, #17117 ) ;
#22405=CARTESIAN_POINT ( 'NONE',  ( -656.9134821118512946, 39.94664452722312831, -2.129547589869284607 ) ) ;
#22417=CARTESIAN_POINT ( 'NONE',  ( -716.9846540392142060, -52.49999999999991473, 52.49999999999999289 ) ) ;
#22423=ORIENTED_EDGE ( 'NONE', *, *, #7424, .F. ) ;
#22432=LINE ( 'NONE', #12562, #15181 ) ;
#22440=DIRECTION ( 'NONE',  ( 1.000000000000000000, 1.836970198721030427E-16, -0.000000000000000000 ) ) ;
#22473=CARTESIAN_POINT ( 'NONE',  ( -210.0000000000000568, 82.50000000000008527, 52.49999999999980105 ) ) ;
#22485=EDGE_LOOP ( 'NONE', ( #8792, #5014 ) ) ;
#22487=CARTESIAN_POINT ( 'NONE',  ( -211.2619052429883482, 0.000000000000000000, -75.00000000000000000 ) ) ;
#22494=CARTESIAN_POINT ( 'NONE',  ( -626.9846540392142060, 105.0000000000000000, 0.000000000000000000 ) ) ;
#22511=CARTESIAN_POINT ( 'NONE',  ( -626.9846540392142060, 90.00000000000000000, -74.99999999999991473 ) ) ;
#22513=EDGE_LOOP ( 'NONE', ( #18604, #3859, #12782, #5974 ) ) ;
#22524=ORIENTED_EDGE ( 'NONE', *, *, #20455, .T. ) ;
#22552=CIRCLE ( 'NONE', #5527, 5.000000000000011546 ) ;
#22581=CIRCLE ( 'NONE', #19180, 30.00000000000000355 ) ;
#22633=CARTESIAN_POINT ( 'NONE',  ( -626.9846540392142060, 28.28427124746186294, -34.99999999999999289 ) ) ;
#22642=CARTESIAN_POINT ( 'NONE',  ( -678.9461782662789346, 90.00000000000000000, -29.99999999999836220 ) ) ;
#22657=CARTESIAN_POINT ( 'NONE',  ( -716.9846540392142060, -52.49999999999972999, -82.49999999999998579 ) ) ;
#22658=EDGE_CURVE ( 'NONE', #25214, #17033, #5917, .T. ) ;
#22666=CARTESIAN_POINT ( 'NONE',  ( -626.9846540392140923, 26.45751311064577749, 30.00000000000005329 ) ) ;
#22673=CARTESIAN_POINT ( 'NONE',  ( -575.0231298121445889, 90.00000000000000000, 29.99999999999825206 ) ) ;
#22675=CARTESIAN_POINT ( 'NONE',  ( -661.4640049366287258, 44.59621196335826454, 6.044506261930657764 ) ) ;
#22679=CARTESIAN_POINT ( 'NONE',  ( -599.8456638329612360, 39.19767421272204189, -22.10842335695227590 ) ) ;
#22684=ORIENTED_EDGE ( 'NONE', *, *, #16318, .F. ) ;
#22694=DIRECTION ( 'NONE',  ( 0.000000000000000000, 0.000000000000000000, 1.000000000000000000 ) ) ;
#22711=VERTEX_POINT ( 'NONE', #6785 ) ;
#22714=DIRECTION ( 'NONE',  ( 0.000000000000000000, 1.000000000000000000, 0.000000000000000000 ) ) ;
#22727=ADVANCED_FACE ( 'NONE', ( #813 ), #4941, .F. ) ;
#22741=ORIENTED_EDGE ( 'NONE', *, *, #26271, .F. ) ;
#22754=VECTOR ( 'NONE', #3242, 1000.000000000000000 ) ;
#22759=FACE_OUTER_BOUND ( 'NONE', #15585, .T. ) ;
#22760=FACE_BOUND ( 'NONE', #16284, .T. ) ;
#22763=CARTESIAN_POINT ( 'NONE',  ( -716.9846540392142060, 66.50000000000009948, 71.50000000000005684 ) ) ;
#22776=CARTESIAN_POINT ( 'NONE',  ( -716.9846540392142060, 52.50000000000007816, -52.49999999999999289 ) ) ;
#22778=ORIENTED_EDGE ( 'NONE', *, *, #24745, .T. ) ;
#22785=ORIENTED_EDGE ( 'NONE', *, *, #24291, .F. ) ;
#22790=AXIS2_PLACEMENT_3D ( 'NONE', #1310, #17276, #15653 ) ;
#22792=DIRECTION ( 'NONE',  ( 0.000000000000000000, 0.000000000000000000, 1.000000000000000000 ) ) ;
#22807=CARTESIAN_POINT ( 'NONE',  ( -641.7033821489691263, 31.87133642205515471, 31.77436929086892903 ) ) ;
#22812=CARTESIAN_POINT ( 'NONE',  ( -593.2054431927236919, 44.05607902751195581, 9.473706874029589997 ) ) ;
#22824=EDGE_CURVE ( 'NONE', #6964, #16641, #17911, .T. ) ;
#22831=CARTESIAN_POINT ( 'NONE',  ( -211.2619052429883482, 0.000000000000000000, 0.000000000000000000 ) ) ;
#22836=EDGE_CURVE ( 'NONE', #25302, #17336, #18661, .T. ) ;
#22850=CARTESIAN_POINT ( 'NONE',  ( -575.0231298121466352, 90.00000000000000000, -30.00000000000202505 ) ) ;
#22889=CARTESIAN_POINT ( 'NONE',  ( -604.2904488564438452, 34.85647621512581651, 19.62648268795706130 ) ) ;
#22898=DIRECTION ( 'NONE',  ( -1.000000000000000000, 0.000000000000000000, 0.000000000000000000 ) ) ;
#22906=AXIS2_PLACEMENT_3D ( 'NONE', #21319, #16925, #25190 ) ;
#22912=LINE ( 'NONE', #14911, #3038 ) ;
#22927=CARTESIAN_POINT ( 'NONE',  ( -656.9692583454861960, 39.98845026487703080, -1.092349456584704948 ) ) ;
#22935=FACE_OUTER_BOUND ( 'NONE', #8170, .T. ) ;
#22941=CARTESIAN_POINT ( 'NONE',  ( -592.0016308006249801, 44.98679260217947018, -1.246943552952227696 ) ) ;
#22945=CARTESIAN_POINT ( 'NONE',  ( -726.9846540392142060, 66.50000000000009948, -61.50000000000004974 ) ) ;
#22957=CARTESIAN_POINT ( 'NONE',  ( -726.9846540392142060, 52.50000000000007816, 52.49999999999999289 ) ) ;
#22975=ADVANCED_FACE ( 'NONE', ( #16922 ), #16788, .F. ) ;
#22985=EDGE_CURVE ( 'NONE', #1721, #2983, #16585, .T. ) ;
#23002=DIRECTION ( 'NONE',  ( 0.000000000000000000, 1.000000000000000000, 0.000000000000000000 ) ) ;
#23008=CIRCLE ( 'NONE', #3439, 5.000000000000004441 ) ;
#23009=VECTOR ( 'NONE', #8823, 1000.000000000000000 ) ;
#23024=AXIS2_PLACEMENT_3D ( 'NONE', #14749, #6503, #6768 ) ;
#23039=CARTESIAN_POINT ( 'NONE',  ( -210.0000000000000284, -52.49999999999992895, -52.49999999999999289 ) ) ;
#23051=AXIS2_PLACEMENT_3D ( 'NONE', #1586, #9689, #15796 ) ;
#23053=CARTESIAN_POINT ( 'NONE',  ( -211.2619052429883482, 0.000000000000000000, 0.000000000000000000 ) ) ;
#23060=DIRECTION ( 'NONE',  ( -1.000000000000000000, 0.000000000000000000, 0.000000000000000000 ) ) ;
#23076=CARTESIAN_POINT ( 'NONE',  ( -661.7304433267322565, 44.80254769115845903, 4.254228907715386754 ) ) ;
#23080=CARTESIAN_POINT ( 'NONE',  ( -626.9846540392142060, 28.28427124746186294, -34.99999999999999289 ) ) ;
#23087=VERTEX_POINT ( 'NONE', #3463 ) ;
#23092=EDGE_CURVE ( 'NONE', #17459, #14871, #15555, .T. ) ;
#23143=ORIENTED_EDGE ( 'NONE', *, *, #18340, .T. ) ;
#23179=ORIENTED_EDGE ( 'NONE', *, *, #22233, .T. ) ;
#23202=ORIENTED_EDGE ( 'NONE', *, *, #7796, .T. ) ;
#23205=CARTESIAN_POINT ( 'NONE',  ( -612.2848868978584278, 31.86264369326284651, -31.78304153250905628 ) ) ;
#23209=CARTESIAN_POINT ( 'NONE',  ( -716.9846540392142060, 66.50000000000009948, 66.50000000000005684 ) ) ;
#23210=VECTOR ( 'NONE', #12299, 1000.000000000000000 ) ;
#23214=ORIENTED_EDGE ( 'NONE', *, *, #19887, .T. ) ;
#23216=CIRCLE ( 'NONE', #24027, 30.00000000000000000 ) ;
#23222=DIRECTION ( 'NONE',  ( 0.000000000000000000, 0.000000000000000000, 1.000000000000000000 ) ) ;
#23241=DIRECTION ( 'NONE',  ( -1.000000000000000000, 0.000000000000000000, 0.000000000000000000 ) ) ;
#23243=VECTOR ( 'NONE', #3738, 1000.000000000000000 ) ;
#23284=CARTESIAN_POINT ( 'NONE',  ( -600.2449649317687772, 37.61268920114236636, 13.74386906026104249 ) ) ;
#23304=CARTESIAN_POINT ( 'NONE',  ( -210.0000000000000284, 52.49999999999988631, -82.49999999999998579 ) ) ;
#23307=VERTEX_POINT ( 'NONE', #13438 ) ;
#23312=CARTESIAN_POINT ( 'NONE',  ( -716.9846540392142060, -66.50000000000001421, 66.50000000000005684 ) ) ;
#23315=EDGE_CURVE ( 'NONE', #15801, #1596, #1470, .T. ) ;
#23323=CYLINDRICAL_SURFACE ( 'NONE', #14263, 30.00000000000000355 ) ;
#23326=FACE_OUTER_BOUND ( 'NONE', #3356, .T. ) ;
#23330=CARTESIAN_POINT ( 'NONE',  ( -631.8022509310842452, 28.60468924217828857, -34.74645141880154142 ) ) ;
#23331=CARTESIAN_POINT ( 'NONE',  ( -726.9846540392142060, 4.898587196589404348E-15, 39.99999999999991473 ) ) ;
#23339=DIRECTION ( 'NONE',  ( -1.000000000000000000, 0.000000000000000000, 0.000000000000000000 ) ) ;
#23364=ORIENTED_EDGE ( 'NONE', *, *, #21498, .T. ) ;
#23372=DIRECTION ( 'NONE',  ( 1.000000000000000000, -0.000000000000000000, -0.000000000000000000 ) ) ;
#23376=CARTESIAN_POINT ( 'NONE',  ( -649.6854717427950163, 34.86078069656281286, -19.61884895816823260 ) ) ;
#23388=DIRECTION ( 'NONE',  ( 0.000000000000000000, 0.000000000000000000, 1.000000000000000000 ) ) ;
#23399=CIRCLE ( 'NONE', #11910, 75.00000000000000000 ) ;
#23408=CARTESIAN_POINT ( 'NONE',  ( -210.0000000000000284, 52.50000000000007816, -52.49999999999999289 ) ) ;
#23411=CARTESIAN_POINT ( 'NONE',  ( -624.9082308837247410, 26.45751311064576683, -30.00000000000002842 ) ) ;
#23417=CARTESIAN_POINT ( 'NONE',  ( -626.9846540392142060, 90.00000000000000000, -60.00000000000000000 ) ) ;
#23419=ORIENTED_EDGE ( 'NONE', *, *, #3969, .T. ) ;
#23431=CIRCLE ( 'NONE', #10695, 75.00000000000000000 ) ;
#23432=LINE ( 'NONE', #7313, #6862 ) ;
#23440=CARTESIAN_POINT ( 'NONE',  ( -575.0231298121445889, 75.00000000000000000, 29.99999999999825206 ) ) ;
#23458=DIRECTION ( 'NONE',  ( 0.000000000000000000, 0.000000000000000000, 1.000000000000000000 ) ) ;
#23489=VERTEX_POINT ( 'NONE', #15442 ) ;
#23493=CARTESIAN_POINT ( 'NONE',  ( -626.9846540392142060, -82.50099999999990530, 0.000000000000000000 ) ) ;
#23497=CARTESIAN_POINT ( 'NONE',  ( -656.1320007476808769, 39.36430177191026303, -7.173594678086772980 ) ) ;
#23525=ADVANCED_FACE ( 'NONE', ( #23326 ), #13084, .T. ) ;
#23537=DIRECTION ( 'NONE',  ( 0.000000000000000000, 1.000000000000000000, 0.000000000000000000 ) ) ;
#23547=ORIENTED_EDGE ( 'NONE', *, *, #8837, .T. ) ;
#23560=DIRECTION ( 'NONE',  ( 0.000000000000000000, 0.000000000000000000, 1.000000000000000000 ) ) ;
#23574=CARTESIAN_POINT ( 'NONE',  ( -644.6425580139975864, 33.33320607737224606, -30.23934288404415938 ) ) ;
#23578=FACE_OUTER_BOUND ( 'NONE', #956, .T. ) ;
#23579=CARTESIAN_POINT ( 'NONE',  ( -620.9980249814747140, 28.88918448956861695, 34.50439121308308899 ) ) ;
#23585=ORIENTED_EDGE ( 'NONE', *, *, #6860, .F. ) ;
#23600=CARTESIAN_POINT ( 'NONE',  ( -626.9846540392142060, 90.00000000000000000, -54.99999999999995026 ) ) ;
#23606=CARTESIAN_POINT ( 'NONE',  ( -716.9846540392142060, 66.50000000000009948, -66.50000000000005684 ) ) ;
#23610=EDGE_LOOP ( 'NONE', ( #7758, #12958 ) ) ;
#23615=DIRECTION ( 'NONE',  ( -0.000000000000000000, 1.000000000000000000, -0.000000000000000000 ) ) ;
#23617=EDGE_CURVE ( 'NONE', #11180, #4752, #23399, .T. ) ;
#23637=AXIS2_PLACEMENT_3D ( 'NONE', #19920, #3694, #13407 ) ;
#23653=DIRECTION ( 'NONE',  ( 0.000000000000000000, 1.000000000000000000, 0.000000000000000000 ) ) ;
#23656=CARTESIAN_POINT ( 'NONE',  ( -597.7037569780933381, 39.46347844285461548, -6.549284831979162114 ) ) ;
#23663=EDGE_LOOP ( 'NONE', ( #7810, #22259 ) ) ;
#23670=ORIENTED_EDGE ( 'NONE', *, *, #24595, .F. ) ;
#23674=ORIENTED_EDGE ( 'NONE', *, *, #23848, .F. ) ;
#23680=DIRECTION ( 'NONE',  ( 0.000000000000000000, -1.000000000000000000, 0.000000000000000000 ) ) ;
#23683=CARTESIAN_POINT ( 'NONE',  ( -626.9846540392097722, 90.00000000000000000, 59.99999999999999289 ) ) ;
#23684=DIRECTION ( 'NONE',  ( 0.000000000000000000, -0.000000000000000000, -1.000000000000000000 ) ) ;
#23698=CARTESIAN_POINT ( 'NONE',  ( -656.4562131466713026, 40.84575396553432824, -18.91241459347874354 ) ) ;
#23702=DIRECTION ( 'NONE',  ( 0.000000000000000000, 1.000000000000000000, 0.000000000000000000 ) ) ;
#23709=ORIENTED_EDGE ( 'NONE', *, *, #19706, .T. ) ;
#23733=AXIS2_PLACEMENT_3D ( 'NONE', #22831, #25224, #609 ) ;
#23772=CIRCLE ( 'NONE', #867, 39.99999999999991473 ) ;
#23778=CARTESIAN_POINT ( 'NONE',  ( -575.0231298121466352, 75.00000000000000000, -35.00000000000203926 ) ) ;
#23789=VERTEX_POINT ( 'NONE', #22473 ) ;
#23827=DIRECTION ( 'NONE',  ( 0.000000000000000000, 1.000000000000000000, 0.000000000000000000 ) ) ;
#23832=VECTOR ( 'NONE', #20127, 1000.000000000000000 ) ;
#23835=CARTESIAN_POINT ( 'NONE',  ( -210.0000000000000284, -66.50000000000001421, -66.50000000000005684 ) ) ;
#23837=ORIENTED_EDGE ( 'NONE', *, *, #12728, .F. ) ;
#23839=CIRCLE ( 'NONE', #19590, 74.99999999999991473 ) ;
#23845=LINE ( 'NONE', #19990, #19955 ) ;
#23848=EDGE_CURVE ( 'NONE', #16014, #15457, #16974, .T. ) ;
#23866=EDGE_CURVE ( 'NONE', #2322, #24112, #7011, .T. ) ;
#23868=CIRCLE ( 'NONE', #25606, 5.000000000000004441 ) ;
#23886=CARTESIAN_POINT ( 'NONE',  ( -210.0000000000000284, 52.50000000000007816, 52.49999999999999289 ) ) ;
#23900=CARTESIAN_POINT ( 'NONE',  ( -626.9846540392142060, 90.00000000000000000, 46.18033988749894547 ) ) ;
#23913=ADVANCED_FACE ( 'NONE', ( #2912 ), #2781, .F. ) ;
#23918=CARTESIAN_POINT ( 'NONE',  ( -210.0000000000000284, 0.000000000000000000, 0.000000000000000000 ) ) ;
#23919=EDGE_LOOP ( 'NONE', ( #243, #13188, #14347, #8064 ) ) ;
#23952=VECTOR ( 'NONE', #15265, 1000.000000000000000 ) ;
#23964=DIRECTION ( 'NONE',  ( 0.000000000000000000, 0.000000000000000000, 1.000000000000000000 ) ) ;
#23971=ORIENTED_EDGE ( 'NONE', *, *, #19855, .T. ) ;
#23989=FACE_BOUND ( 'NONE', #21552, .T. ) ;
#24007=CARTESIAN_POINT ( 'NONE',  ( -626.9846540392142060, 75.00000000000000000, -54.99999999999995026 ) ) ;
#24027=AXIS2_PLACEMENT_3D ( 'NONE', #16756, #5060, #14759 ) ;
#24029=VERTEX_POINT ( 'NONE', #20999 ) ;
#24034=AXIS2_PLACEMENT_3D ( 'NONE', #4208, #4466, #8440 ) ;
#24036=AXIS2_PLACEMENT_3D ( 'NONE', #1684, #3813, #19505 ) ;
#24038=ORIENTED_EDGE ( 'NONE', *, *, #11099, .T. ) ;
#24064=VERTEX_POINT ( 'NONE', #11145 ) ;
#24077=CIRCLE ( 'NONE', #16853, 5.000000000000004441 ) ;
#24084=FACE_BOUND ( 'NONE', #7020, .T. ) ;
#24088=FACE_OUTER_BOUND ( 'NONE', #6437, .T. ) ;
#24098=LINE ( 'NONE', #7989, #12312 ) ;
#24100=DIRECTION ( 'NONE',  ( 0.000000000000000000, 0.000000000000000000, 1.000000000000000000 ) ) ;
#24107=ORIENTED_EDGE ( 'NONE', *, *, #6969, .T. ) ;
#24110=EDGE_CURVE ( 'NONE', #18109, #11822, #8929, .T. ) ;
#24112=VERTEX_POINT ( 'NONE', #4906 ) ;
#24113=ORIENTED_EDGE ( 'NONE', *, *, #18653, .T. ) ;
#24114=CARTESIAN_POINT ( 'NONE',  ( -210.0000000000000284, -71.50000000000002842, 66.50000000000005684 ) ) ;
#24118=EDGE_CURVE ( 'NONE', #3746, #3578, #23772, .T. ) ;
#24123=CARTESIAN_POINT ( 'NONE',  ( -635.0400797919774050, 27.64234391852529171, -28.91503648664665960 ) ) ;
#24134=PLANE ( 'NONE',  #4516 ) ;
#24153=DIRECTION ( 'NONE',  ( 0.000000000000000000, 0.000000000000000000, -1.000000000000000000 ) ) ;
#24156=DIRECTION ( 'NONE',  ( 0.000000000000000000, 0.000000000000000000, 1.000000000000000000 ) ) ;
#24167=ORIENTED_EDGE ( 'NONE', *, *, #15616, .F. ) ;
#24180=AXIS2_PLACEMENT_3D ( 'NONE', #23493, #23615, #3020 ) ;
#24201=ORIENTED_EDGE ( 'NONE', *, *, #26318, .F. ) ;
#24202=ORIENTED_EDGE ( 'NONE', *, *, #5343, .F. ) ;
#24208=VECTOR ( 'NONE', #1266, 1000.000000000000000 ) ;
#24209=ADVANCED_FACE ( 'NONE', ( #5873 ), #8257, .F. ) ;
#24229=CIRCLE ( 'NONE', #1282, 5.000000000000011546 ) ;
#24230=CARTESIAN_POINT ( 'NONE',  ( -716.9846540392142060, -66.50000000000001421, -66.50000000000005684 ) ) ;
#24237=EDGE_LOOP ( 'NONE', ( #10927, #2518, #21176, #5357 ) ) ;
#24239=DIRECTION ( 'NONE',  ( 1.000000000000000000, -0.000000000000000000, -0.000000000000000000 ) ) ;
#24246=CARTESIAN_POINT ( 'NONE',  ( -210.0000000000000284, 66.50000000000009948, -66.50000000000005684 ) ) ;
#24248=ORIENTED_EDGE ( 'NONE', *, *, #4789, .T. ) ;
#24261=DIRECTION ( 'NONE',  ( 0.000000000000000000, 0.000000000000000000, 1.000000000000000000 ) ) ;
#24263=ADVANCED_FACE ( 'NONE', ( #2154 ), #15605, .F. ) ;
#24268=AXIS2_PLACEMENT_3D ( 'NONE', #3328, #11427, #5204 ) ;
#24286=AXIS2_PLACEMENT_3D ( 'NONE', #13397, #15009, #19514 ) ;
#24291=EDGE_CURVE ( 'NONE', #2553, #5353, #24098, .T. ) ;
#24298=DIRECTION ( 'NONE',  ( 1.000000000000000000, -0.000000000000000000, -0.000000000000000000 ) ) ;
#24303=EDGE_CURVE ( 'NONE', #9693, #1564, #18, .T. ) ;
#24341=ORIENTED_EDGE ( 'NONE', *, *, #22658, .F. ) ;
#24364=FACE_BOUND ( 'NONE', #13059, .T. ) ;
#24366=FACE_OUTER_BOUND ( 'NONE', #21271, .T. ) ;
#24373=EDGE_LOOP ( 'NONE', ( #9636, #9829, #19799, #2198 ) ) ;
#24393=CARTESIAN_POINT ( 'NONE',  ( -649.4031135302850544, 34.67746518522525179, 19.94086391362369781 ) ) ;
#24396=DIRECTION ( 'NONE',  ( 0.000000000000000000, 1.000000000000000000, 0.000000000000000000 ) ) ;
#24411=EDGE_LOOP ( 'NONE', ( #8705, #14315 ) ) ;
#24417=DIRECTION ( 'NONE',  ( -1.000000000000000000, -1.836970198721030181E-16, 0.000000000000000000 ) ) ;
#24418=CARTESIAN_POINT ( 'NONE',  ( -716.9846540392142060, -52.49999999999991473, 52.49999999999999289 ) ) ;
#24427=CARTESIAN_POINT ( 'NONE',  ( -210.0000000000000000, -82.49999999999991473, -52.49999999999977973 ) ) ;
#24445=ADVANCED_FACE ( 'NONE', ( #9370 ), #22113, .T. ) ;
#24468=AXIS2_PLACEMENT_3D ( 'NONE', #420, #24771, #24903 ) ;
#24477=ORIENTED_EDGE ( 'NONE', *, *, #15793, .F. ) ;
#24482=AXIS2_PLACEMENT_3D ( 'NONE', #15448, #3228, #11452 ) ;
#24499=FACE_BOUND ( 'NONE', #16244, .T. ) ;
#24505=DIRECTION ( 'NONE',  ( 0.000000000000000000, 1.000000000000000000, 0.000000000000000000 ) ) ;
#24515=ORIENTED_EDGE ( 'NONE', *, *, #10595, .F. ) ;
#24520=AXIS2_PLACEMENT_3D ( 'NONE', #13831, #5599, #14109 ) ;
#24530=CARTESIAN_POINT ( 'NONE',  ( -656.7096227442339114, 39.79407741042334834, -4.181560688537802051 ) ) ;
#24538=CARTESIAN_POINT ( 'NONE',  ( -210.0000000000000284, 66.50000000000009948, -66.50000000000005684 ) ) ;
#24542=AXIS2_PLACEMENT_3D ( 'NONE', #8897, #15142, #15013 ) ;
#24550=ORIENTED_EDGE ( 'NONE', *, *, #16145, .T. ) ;
#24586=AXIS2_PLACEMENT_3D ( 'NONE', #3092, #17685, #23684 ) ;
#24595=EDGE_CURVE ( 'NONE', #3578, #21399, #22248, .T. ) ;
#24600=EDGE_CURVE ( 'NONE', #26151, #5117, #9334, .T. ) ;
#24603=ORIENTED_EDGE ( 'NONE', *, *, #9770, .F. ) ;
#24612=ORIENTED_EDGE ( 'NONE', *, *, #9011, .F. ) ;
#24632=LINE ( 'NONE', #6390, #9639 ) ;
#24635=ADVANCED_FACE ( 'NONE', ( #685 ), #25039, .F. ) ;
#24636=ORIENTED_EDGE ( 'NONE', *, *, #25270, .T. ) ;
#24638=DIRECTION ( 'NONE',  ( -1.000000000000000000, 0.000000000000000000, 0.000000000000000000 ) ) ;
#24649=ORIENTED_EDGE ( 'NONE', *, *, #23617, .T. ) ;
#24658=VECTOR ( 'NONE', #18235, 1000.000000000000000 ) ;
#24661=CARTESIAN_POINT ( 'NONE',  ( -629.5670837480076898, 26.57842901870468211, 29.89303253829147167 ) ) ;
#24667=CARTESIAN_POINT ( 'NONE',  ( -200.0000000000000000, -69.99999999999998579, 8.572527594031471415E-15 ) ) ;
#24669=DIRECTION ( 'NONE',  ( 0.000000000000000000, 1.000000000000000000, 0.000000000000000000 ) ) ;
#24671=CARTESIAN_POINT ( 'NONE',  ( -644.6571494263627073, 33.34084698429052196, 30.23100662976579045 ) ) ;
#24675=CARTESIAN_POINT ( 'NONE',  ( -618.7358282227124846, 29.45763196998035127, -34.01907996191106065 ) ) ;
#24689=EDGE_CURVE ( 'NONE', #25953, #4298, #12737, .T. ) ;
#24691=VECTOR ( 'NONE', #12502, 1000.000000000000000 ) ;
#24726=AXIS2_PLACEMENT_3D ( 'NONE', #7698, #7964, #22222 ) ;
#24734=DIRECTION ( 'NONE',  ( 0.000000000000000000, 1.000000000000000000, 0.000000000000000000 ) ) ;
#24745=EDGE_CURVE ( 'NONE', #25083, #2152, #16125, .T. ) ;
#24746=ORIENTED_EDGE ( 'NONE', *, *, #26072, .T. ) ;
#24771=DIRECTION ( 'NONE',  ( -1.000000000000000000, 0.000000000000000000, 0.000000000000000000 ) ) ;
#24774=SHAPE_REPRESENTATION ( 'Pump housing', ( #21058 ), #9559 ) ;
#24780=CARTESIAN_POINT ( 'NONE',  ( -200.0000000000000000, 71.50000000000011369, -66.50000000000005684 ) ) ;
#24784=EDGE_CURVE ( 'NONE', #5675, #12661, #4684, .T. ) ;
#24785=EDGE_LOOP ( 'NONE', ( #11218, #22356, #11548, #2064, #15508 ) ) ;
#24803=FACE_OUTER_BOUND ( 'NONE', #22513, .T. ) ;
#24805=CARTESIAN_POINT ( 'NONE',  ( -648.3028445202884313, 35.38721658766822031, 27.84362906246311553 ) ) ;
#24809=CARTESIAN_POINT ( 'NONE',  ( -624.5354243231303144, 28.28427124746188781, -34.99999999999999289 ) ) ;
#24813=ORIENTED_EDGE ( 'NONE', *, *, #2404, .T. ) ;
#24816=CARTESIAN_POINT ( 'NONE',  ( -716.9846540392142060, -66.50000000000001421, -66.50000000000005684 ) ) ;
#24870=CARTESIAN_POINT ( 'NONE',  ( -716.9846540392142060, -66.50000000000001421, -61.50000000000006395 ) ) ;
#24890=CARTESIAN_POINT ( 'NONE',  ( -597.2601520101716233, 39.79372847804995672, 4.185400860730163153 ) ) ;
#24903=DIRECTION ( 'NONE',  ( 0.000000000000000000, 0.000000000000000000, 1.000000000000000000 ) ) ;
#24912=VECTOR ( 'NONE', #5185, 1000.000000000000000 ) ;
#24917=ORIENTED_EDGE ( 'NONE', *, *, #20785, .T. ) ;
#24923=AXIS2_PLACEMENT_3D ( 'NONE', #9521, #7390, #15501 ) ;
#24926=VECTOR ( 'NONE', #16518, 1000.000000000000000 ) ;
#24928=DIRECTION ( 'NONE',  ( 1.000000000000000000, -0.000000000000000000, -0.000000000000000000 ) ) ;
#24939=FACE_OUTER_BOUND ( 'NONE', #187, .T. ) ;
#24941=CARTESIAN_POINT ( 'NONE',  ( -210.0000000000000284, -69.99999999999998579, 8.572527594031471415E-15 ) ) ;
#24948=CARTESIAN_POINT ( 'NONE',  ( -599.4962176833719241, 39.44053679066730922, -21.67249732420721031 ) ) ;
#24951=ADVANCED_FACE ( 'NONE', ( #14632 ), #16765, .F. ) ;
#24956=ORIENTED_EDGE ( 'NONE', *, *, #18731, .F. ) ;
#24958=LINE ( 'NONE', #4862, #25328 ) ;
#24960=AXIS2_PLACEMENT_3D ( 'NONE', #19035, #22898, #8789 ) ;
#25033=FACE_BOUND ( 'NONE', #23663, .T. ) ;
#25036=ORIENTED_EDGE ( 'NONE', *, *, #20398, .T. ) ;
#25039=CYLINDRICAL_SURFACE ( 'NONE', #17394, 5.000000000000004441 ) ;
#25042=ADVANCED_FACE ( 'NONE', ( #8657 ), #6654, .T. ) ;
#25063=DIRECTION ( 'NONE',  ( -1.000000000000000000, -1.836970198721030181E-16, 0.000000000000000000 ) ) ;
#25065=VECTOR ( 'NONE', #17506, 1000.000000000000000 ) ;
#25083=VERTEX_POINT ( 'NONE', #22511 ) ;
#25107=LINE ( 'NONE', #12985, #26196 ) ;
#25121=EDGE_CURVE ( 'NONE', #26265, #23307, #22552, .T. ) ;
#25134=DIRECTION ( 'NONE',  ( 0.000000000000000000, -1.000000000000000000, 0.000000000000000000 ) ) ;
#25136=AXIS2_PLACEMENT_3D ( 'NONE', #21637, #21514, #23388 ) ;
#25138=ORIENTED_EDGE ( 'NONE', *, *, #1126, .T. ) ;
#25187=DIRECTION ( 'NONE',  ( 1.000000000000000000, -0.000000000000000000, -0.000000000000000000 ) ) ;
#25189=FACE_OUTER_BOUND ( 'NONE', #19427, .T. ) ;
#25190=DIRECTION ( 'NONE',  ( 0.000000000000000000, 0.000000000000000000, 1.000000000000000000 ) ) ;
#25195=CIRCLE ( 'NONE', #18368, 5.000000000000095035 ) ;
#25204=CARTESIAN_POINT ( 'NONE',  ( -654.4889232350201382, 39.44889917058262796, 21.67367656778695917 ) ) ;
#25205=DIRECTION ( 'NONE',  ( -1.000000000000000000, -1.836970198721030181E-16, 0.000000000000000000 ) ) ;
#25209=CARTESIAN_POINT ( 'NONE',  ( -592.0438061236260410, 44.95394254848083904, 2.361432597285608725 ) ) ;
#25214=VERTEX_POINT ( 'NONE', #7753 ) ;
#25224=DIRECTION ( 'NONE',  ( 1.000000000000000000, -0.000000000000000000, -0.000000000000000000 ) ) ;
#25236=ORIENTED_EDGE ( 'NONE', *, *, #12545, .F. ) ;
#25239=DIRECTION ( 'NONE',  ( 0.000000000000000000, -1.000000000000000000, 0.000000000000000000 ) ) ;
#25265=ORIENTED_EDGE ( 'NONE', *, *, #6208, .F. ) ;
#25270=EDGE_CURVE ( 'NONE', #7651, #16549, #25942, .T. ) ;
#25281=CARTESIAN_POINT ( 'NONE',  ( -716.9846540392142060, 0.000000000000000000, 0.000000000000000000 ) ) ;
#25285=CARTESIAN_POINT ( 'NONE',  ( -604.6053156620442905, 34.65218274561313905, 19.98475300726100201 ) ) ;
#25292=DIRECTION ( 'NONE',  ( 0.000000000000000000, 0.000000000000000000, 1.000000000000000000 ) ) ;
#25295=EDGE_LOOP ( 'NONE', ( #19423, #18276, #25910, #9476 ) ) ;
#25302=VERTEX_POINT ( 'NONE', #14809 ) ;
#25303=ORIENTED_EDGE ( 'NONE', *, *, #1200, .F. ) ;
#25310=AXIS2_PLACEMENT_3D ( 'NONE', #4052, #5631, #14803 ) ;
#25328=VECTOR ( 'NONE', #6704, 1000.000000000000000 ) ;
#25331=CARTESIAN_POINT ( 'NONE',  ( -641.7036307566764890, 31.87148209193353665, -31.77421052347908415 ) ) ;
#25336=CARTESIAN_POINT ( 'NONE',  ( -619.2650551519561759, 29.31345288821323791, 34.14316883558051074 ) ) ;
#25352=VECTOR ( 'NONE', #15912, 1000.000000000000000 ) ;
#25353=CARTESIAN_POINT ( 'NONE',  ( -626.9846540392142060, 26.45751311064579880, -30.00000000000005329 ) ) ;
#25360=EDGE_CURVE ( 'NONE', #12649, #18983, #20434, .T. ) ;
#25365=VECTOR ( 'NONE', #1094, 1000.000000000000000 ) ;
#25370=ADVANCED_FACE ( 'NONE', ( #13583 ), #17705, .F. ) ;
#25373=CARTESIAN_POINT ( 'NONE',  ( -210.0000000000000284, -82.49999999999990052, 52.49999999999977263 ) ) ;
#25380=CARTESIAN_POINT ( 'NONE',  ( -642.9364793054111260, 30.88727062095852816, -25.42494723607509499 ) ) ;
#25392=AXIS2_PLACEMENT_3D ( 'NONE', #25281, #1188, #7289 ) ;
#25411=DIRECTION ( 'NONE',  ( 0.000000000000000000, 1.000000000000000000, 0.000000000000000000 ) ) ;
#25414=CARTESIAN_POINT ( 'NONE',  ( -624.9005621318009389, 26.45751311064577749, 30.00000000000004974 ) ) ;
#25417=EDGE_CURVE ( 'NONE', #15830, #14785, #12759, .T. ) ;
#25432=ORIENTED_EDGE ( 'NONE', *, *, #17354, .T. ) ;
#25435=DIRECTION ( 'NONE',  ( -1.000000000000000000, -1.836970198721030427E-16, 0.000000000000000000 ) ) ;
#25437=ORIENTED_EDGE ( 'NONE', *, *, #24118, .F. ) ;
#25439=LINE ( 'NONE', #25689, #10271 ) ;
#25444=DIRECTION ( 'NONE',  ( 0.000000000000000000, 1.000000000000000000, 0.000000000000000000 ) ) ;
#25452=DIRECTION ( 'NONE',  ( 0.000000000000000000, 0.000000000000000000, 1.000000000000000000 ) ) ;
#25460=LINE ( 'NONE', #1107, #22359 ) ;
#25469=EDGE_LOOP ( 'NONE', ( #21073, #11687, #4030, #627 ) ) ;
#25474=CONICAL_SURFACE ( 'NONE', #23733, 75.00000000000000000, 0.4944367829892072352 ) ;
#25477=AXIS2_PLACEMENT_3D ( 'NONE', #1100, #979, #9210 ) ;
#25499=CARTESIAN_POINT ( 'NONE',  ( 0.000000000000000000, 5.510910596163085611E-15, 44.99999999999997158 ) ) ;
#25502=DIRECTION ( 'NONE',  ( 0.000000000000000000, 0.000000000000000000, -1.000000000000000000 ) ) ;
#25506=CARTESIAN_POINT ( 'NONE',  ( -655.4136578433802924, 38.83551722856093136, -9.594100677173759806 ) ) ;
#25521=DIRECTION ( 'NONE',  ( 1.000000000000000000, 1.836970198721030427E-16, -0.000000000000000000 ) ) ;
#25528=FACE_OUTER_BOUND ( 'NONE', #1118, .T. ) ;
#25531=VECTOR ( 'NONE', #4490, 1000.000000000000000 ) ;
#25536=CYLINDRICAL_SURFACE ( 'NONE', #23637, 5.000000000000018652 ) ;
#25541=FACE_OUTER_BOUND ( 'NONE', #5541, .T. ) ;
#25542=CARTESIAN_POINT ( 'NONE',  ( -608.6692201736730112, 32.15154313405594877, -23.83432366117598633 ) ) ;
#25546=AXIS2_PLACEMENT_3D ( 'NONE', #584, #4843, #451 ) ;
#25560=AXIS2_PLACEMENT_3D ( 'NONE', #12993, #23241, #18984 ) ;
#25587=CARTESIAN_POINT ( 'NONE',  ( -657.0499062528585910, 41.27686082678435042, -17.95486116563373002 ) ) ;
#25599=EDGE_LOOP ( 'NONE', ( #12833, #2867, #20645, #5194 ) ) ;
#25606=AXIS2_PLACEMENT_3D ( 'NONE', #23835, #3236, #11093 ) ;
#25610=CYLINDRICAL_SURFACE ( 'NONE', #10066, 4.999999999999997335 ) ;
#25622=DIRECTION ( 'NONE',  ( -1.000000000000000000, -1.836970198721030181E-16, 0.000000000000000000 ) ) ;
#25625=EDGE_LOOP ( 'NONE', ( #7731, #383 ) ) ;
#25630=CYLINDRICAL_SURFACE ( 'NONE', #24180, 30.00000000000004974 ) ;
#25645=DIRECTION ( 'NONE',  ( 1.000000000000000000, -0.000000000000000000, -0.000000000000000000 ) ) ;
#25661=CARTESIAN_POINT ( 'NONE',  ( -626.9846540392142060, 95.00000000000000000, -34.99999999999999289 ) ) ;
#25664=FACE_OUTER_BOUND ( 'NONE', #1531, .T. ) ;
#25667=CARTESIAN_POINT ( 'NONE',  ( -613.5029046138316744, 29.69186907203735259, -26.80434989160759329 ) ) ;
#25681=ORIENTED_EDGE ( 'NONE', *, *, #12092, .T. ) ;
#25689=CARTESIAN_POINT ( 'NONE',  ( -200.0000000000000000, -52.49999999999991473, 82.49999999999998579 ) ) ;
#25708=CARTESIAN_POINT ( 'NONE',  ( -661.4804418431098156, 44.60892237560697993, -5.950252532928291593 ) ) ;
#25725=CARTESIAN_POINT ( 'NONE',  ( -716.9846540392142060, -82.49999999999991473, 52.49999999999977263 ) ) ;
#25729=AXIS2_PLACEMENT_3D ( 'NONE', #10294, #10161, #8159 ) ;
#25771=CYLINDRICAL_SURFACE ( 'NONE', #24036, 5.000000000000004441 ) ;
#25792=AXIS2_PLACEMENT_3D ( 'NONE', #3068, #13173, #6916 ) ;
#25803=ADVANCED_BREP_SHAPE_REPRESENTATION ( '', ( #25811, #21058 ), #9559 ) ;
#25808=DIRECTION ( 'NONE',  ( 0.000000000000000000, -1.000000000000000000, 0.000000000000000000 ) ) ;
#25811=MANIFOLD_SOLID_BREP ( 'Boss-Extrude13', #3243 ) ;
#25812=EDGE_LOOP ( 'NONE', ( #8805, #19211, #158, #23837, #20515 ) ) ;
#25820=DIRECTION ( 'NONE',  ( 0.8802361161597901384, 5.811389476877143134E-17, 0.4745359626076072757 ) ) ;
#25821=EDGE_CURVE ( 'NONE', #5675, #9962, #4295, .T. ) ;
#25827=EDGE_CURVE ( 'NONE', #10128, #25302, #12385, .T. ) ;
#25834=EDGE_CURVE ( 'NONE', #13991, #19296, #24229, .T. ) ;
#25837=EDGE_CURVE ( 'NONE', #15268, #17459, #11893, .T. ) ;
#25838=CARTESIAN_POINT ( 'NONE',  ( -626.9846540392142060, 90.00000000000000000, 0.000000000000000000 ) ) ;
#25847=LINE ( 'NONE', #13843, #9401 ) ;
#25851=ORIENTED_EDGE ( 'NONE', *, *, #9629, .F. ) ;
#25855=ORIENTED_EDGE ( 'NONE', *, *, #5343, .T. ) ;
#25870=CARTESIAN_POINT ( 'NONE',  ( -726.9846540392142060, -82.49999999999991473, 52.49999999999977263 ) ) ;
#25904=AXIS2_PLACEMENT_3D ( 'NONE', #20248, #4023, #5385 ) ;
#25910=ORIENTED_EDGE ( 'NONE', *, *, #15882, .T. ) ;
#25932=CARTESIAN_POINT ( 'NONE',  ( -598.0754867585920920, 39.18842370550271426, -8.032326897551609335 ) ) ;
#25942=CIRCLE ( 'NONE', #11073, 46.18033988749894547 ) ;
#25953=VERTEX_POINT ( 'NONE', #823 ) ;
#25987=EDGE_LOOP ( 'NONE', ( #17639, #1599 ) ) ;
#25989=CARTESIAN_POINT ( 'NONE',  ( -265.6482238768269326, 0.000000000000000000, 0.000000000000000000 ) ) ;
#26011=CARTESIAN_POINT ( 'NONE',  ( -210.0000000000000284, 0.000000000000000000, -69.99999999999998579 ) ) ;
#26012=FACE_BOUND ( 'NONE', #13517, .T. ) ;
#26038=DIRECTION ( 'NONE',  ( -1.000000000000000000, 0.000000000000000000, 0.000000000000000000 ) ) ;
#26052=ORIENTED_EDGE ( 'NONE', *, *, #3424, .T. ) ;
#26054=CARTESIAN_POINT ( 'NONE',  ( -716.9846540392142060, -66.50000000000001421, -61.50000000000006395 ) ) ;
#26072=EDGE_CURVE ( 'NONE', #3167, #7987, #21676, .T. ) ;
#26089=CARTESIAN_POINT ( 'NONE',  ( -726.9846540392142060, -66.50000000000001421, -66.50000000000005684 ) ) ;
#26132=CARTESIAN_POINT ( 'NONE',  ( -626.9846540392142060, 95.00000000000000000, -30.00000000000005684 ) ) ;
#26151=VERTEX_POINT ( 'NONE', #17166 ) ;
#26163=DIRECTION ( 'NONE',  ( 0.000000000000000000, 1.000000000000000000, 0.000000000000000000 ) ) ;
#26177=EDGE_CURVE ( 'NONE', #1760, #567, #12555, .T. ) ;
#26196=VECTOR ( 'NONE', #10994, 1000.000000000000000 ) ;
#26204=DIRECTION ( 'NONE',  ( 0.000000000000000000, -1.000000000000000000, 0.000000000000000000 ) ) ;
#26214=ORIENTED_EDGE ( 'NONE', *, *, #3626, .F. ) ;
#26245=CYLINDRICAL_SURFACE ( 'NONE', #6411, 4.999999999999997335 ) ;
#26252=ORIENTED_EDGE ( 'NONE', *, *, #20692, .T. ) ;
#26265=VERTEX_POINT ( 'NONE', #12681 ) ;
#26271=EDGE_CURVE ( 'NONE', #18983, #12649, #7362, .T. ) ;
#26275=CARTESIAN_POINT ( 'NONE',  ( -631.0906524188512776, 26.75521908153718798, -29.73521811825018801 ) ) ;
#26280=DIRECTION ( 'NONE',  ( -1.000000000000000000, 0.000000000000000000, 0.000000000000000000 ) ) ;
#26318=EDGE_CURVE ( 'NONE', #21399, #87, #10433, .T. ) ;
#26368=COLOUR_RGB('Dark Blue',0.08,0.2,0.34);
#26369=FILL_AREA_STYLE_COLOUR('',#26368);
#26370=FILL_AREA_STYLE('',(#26369));
#26371=SURFACE_STYLE_FILL_AREA(#26370);
#26372=SURFACE_SIDE_STYLE('',(#26371));
#26373=SURFACE_STYLE_USAGE(.BOTH.,#26372);
#26374=PRESENTATION_STYLE_ASSIGNMENT((#26373));
ENDSEC;
END-ISO-10303-21;
